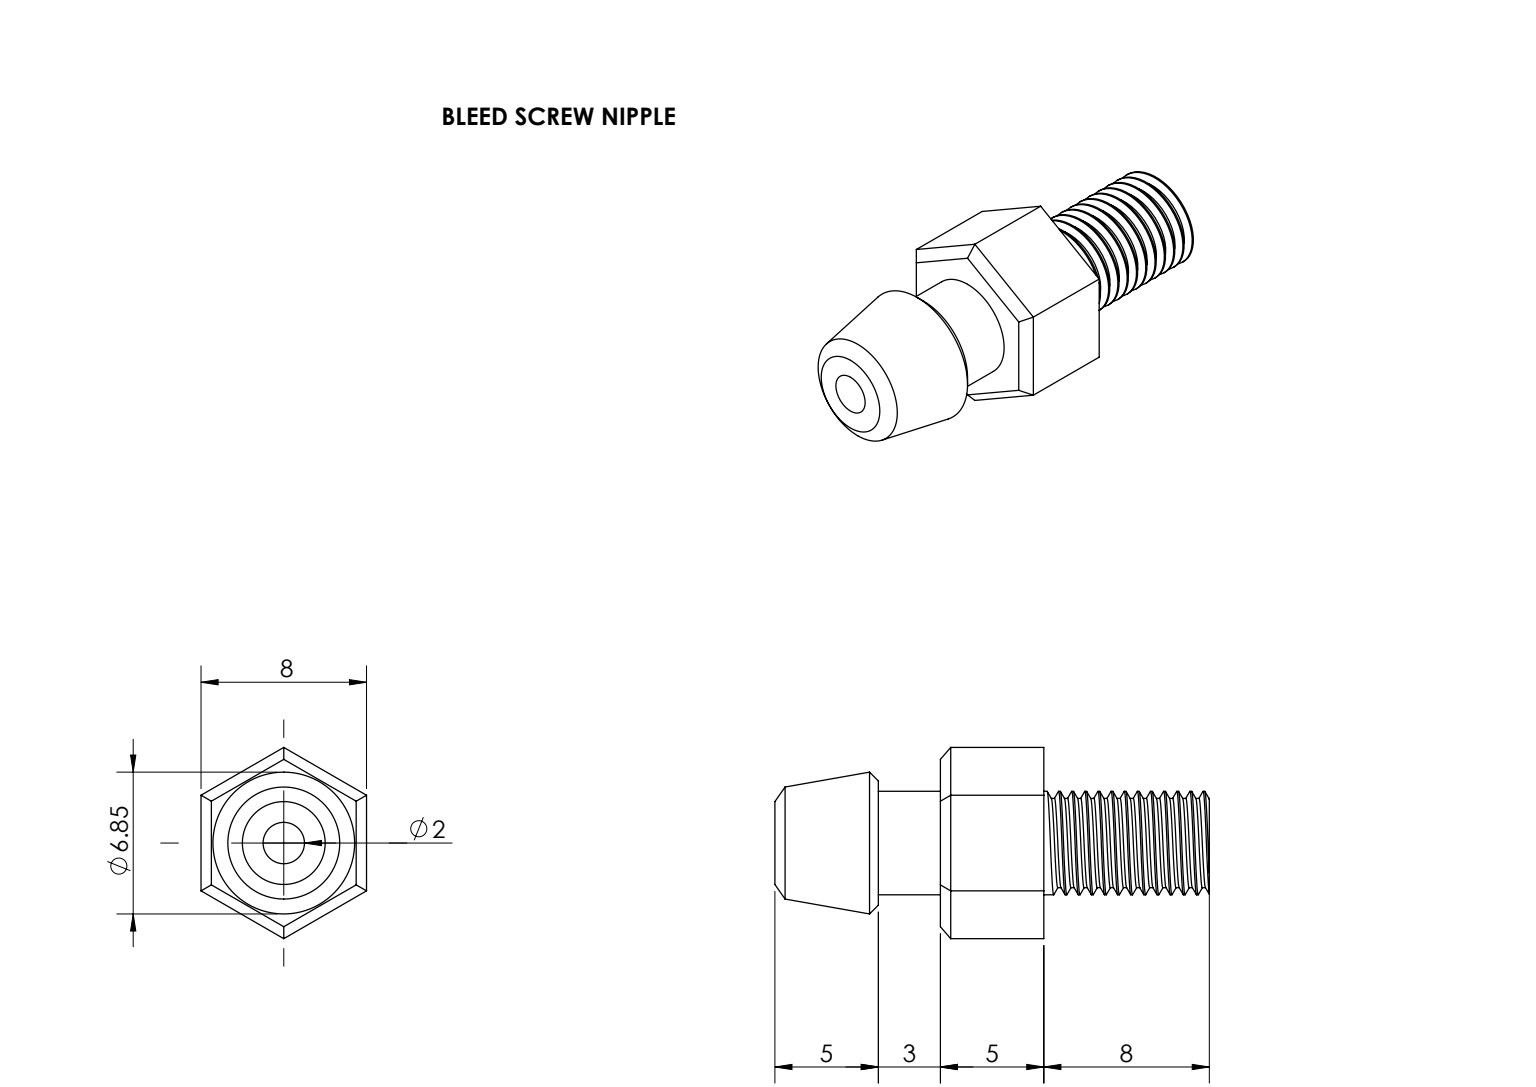
ISO-10303-21;
HEADER;
FILE_DESCRIPTION (('STEP AP214'),
    '1' );
FILE_NAME ('Bleed Screw Nipple.step',
    '2026-09-24T10:28:59',
    ( '' ),
    ( '' ),
    'SwSTEP 2.0',
    'SolidWorks 2026',
    '' );
FILE_SCHEMA (( 'AUTOMOTIVE_DESIGN' ));
ENDSEC;

DATA;
#2=CARTESIAN_POINT ( 'NONE',  ( 28.76238721243587193, -5.825490297734302381, -3.627061608673667781 ) ) ;
#3=CARTESIAN_POINT ( 'NONE',  ( 28.60033944477555323, -4.591072787911525843, -8.283357778048662468 ) ) ;
#4=FACE_OUTER_BOUND ( 'NONE', #16848, .T. ) ;
#16=CARTESIAN_POINT ( 'NONE',  ( 29.62036837594175154, -3.214238380052812261, -3.627061608673662896 ) ) ;
#18=ORIENTED_EDGE ( 'NONE', *, *, #8443, .T. ) ;
#21=CARTESIAN_POINT ( 'NONE',  ( 32.63137222500256485, -6.623491938275930302, -6.453230759126470595 ) ) ;
#34=CONICAL_SURFACE ( 'NONE', #10154, 3.500000000000004885, 0.1745329251994333364 ) ;
#35=CARTESIAN_POINT ( 'NONE',  ( 26.41562710823574278, -3.600346414165641828, -7.939653947423660263 ) ) ;
#38=ORIENTED_EDGE ( 'NONE', *, *, #3823, .T. ) ;
#44=VECTOR ( 'NONE', #8259, 1000.000000000000227 ) ;
#61=AXIS2_PLACEMENT_3D ( 'NONE', #16473, #4043, #10648 ) ;
#72=CARTESIAN_POINT ( 'NONE',  ( 25.86833963875586306, -3.039313213345869791, -4.705209693361160461 ) ) ;
#74=CARTESIAN_POINT ( 'NONE',  ( 29.12189622942009493, -1.620608325512071568, -5.783357778048658027 ) ) ;
#76=CARTESIAN_POINT ( 'NONE',  ( 31.70371634254663817, -2.036456781249897485, -4.533357778048659803 ) ) ;
#81=CARTESIAN_POINT ( 'NONE',  ( 29.62036837594175154, -3.214238380052812261, -3.627061608673662896 ) ) ;
#82=VERTEX_POINT ( 'NONE', #13166 ) ;
#84=CARTESIAN_POINT ( 'NONE',  ( 27.88665588685489993, -3.423116496867954162, -3.627061608673662008 ) ) ;
#95=CARTESIAN_POINT ( 'NONE',  ( 27.62849893492243325, -6.589071975465733644, -4.705209693361168455 ) ) ;
#97=LINE ( 'NONE', #5605, #15979 ) ;
#109=CARTESIAN_POINT ( 'NONE',  ( 26.84461768998868436, -2.294720455324902542, -5.783357778048658915 ) ) ;
#111=PLANE ( 'NONE',  #4436 ) ;
#119=ORIENTED_EDGE ( 'NONE', *, *, #5679, .T. ) ;
#123=CARTESIAN_POINT ( 'NONE',  ( 31.90644508241650357, -6.373472726347483963, -7.033357778048666908 ) ) ;
#135=ORIENTED_EDGE ( 'NONE', *, *, #7750, .F. ) ;
#150=CARTESIAN_POINT ( 'NONE',  ( 31.92138306490751987, -2.737139032229836566, -3.283357778048662023 ) ) ;
#160=CARTESIAN_POINT ( 'NONE',  ( 26.52522735095806894, -6.721994413439005278, -4.705209693361169343 ) ) ;
#161=CARTESIAN_POINT ( 'NONE',  ( 33.50243880635947846, -1.482387629897225390, -5.783357778048663356 ) ) ;
#162=CARTESIAN_POINT ( 'NONE',  ( 27.92859066579839222, -3.218191664895003967, -8.283357778048658915 ) ) ;
#166=CARTESIAN_POINT ( 'NONE',  ( 31.30154412293507349, -3.011689903141150815, -7.939653947423660263 ) ) ;
#168=CARTESIAN_POINT ( 'NONE',  ( 28.28502977505876359, -2.748149777785362957, -6.861505862736158257 ) ) ;
#179=CARTESIAN_POINT ( 'NONE',  ( 29.35841309260160159, -6.680460261459264970, -4.533357778048668685 ) ) ;
#180=CARTESIAN_POINT ( 'NONE',  ( 29.51982165028991645, -6.361204938940122844, -4.705209693361168455 ) ) ;
#191=CARTESIAN_POINT ( 'NONE',  ( 39.34669483983374505, -6.862522726337943801, -6.650911402496568314 ) ) ;
#193=CARTESIAN_POINT ( 'NONE',  ( 27.60205212784272177, -2.830435096530727446, -4.705209693361161349 ) ) ;
#195=ORIENTED_EDGE ( 'NONE', *, *, #15251, .T. ) ;
#209=CARTESIAN_POINT ( 'NONE',  ( 42.20068782821381603, -5.470578387159230616, -5.783357778048662468 ) ) ;
#212=CARTESIAN_POINT ( 'NONE',  ( 33.55383270609817714, -5.448088258586239796, -3.283357778048667797 ) ) ;
#214=CARTESIAN_POINT ( 'NONE',  ( 31.61111609099199171, -1.710254666422835745, -5.783357778048662468 ) ) ;
#220=DIRECTION ( 'NONE',  ( 0.9928203230275512992, 0.1196152422706610319, 9.614813431917826478E-17 ) ) ;
#245=ORIENTED_EDGE ( 'NONE', *, *, #2656, .T. ) ;
#247=DIRECTION ( 'NONE',  ( -0.9928203230275512992, -0.1196152422706610319, -9.614813431917826478E-17 ) ) ;
#252=CYLINDRICAL_SURFACE ( 'NONE', #8155, 1.000000000000000000 ) ;
#255=CARTESIAN_POINT ( 'NONE',  ( 31.11087420047036289, -5.742416513891037688, -3.283357778048667797 ) ) ;
#260=CARTESIAN_POINT ( 'NONE',  ( 32.77257290155422709, -2.834459985843461816, -3.627061608673662896 ) ) ;
#262=CARTESIAN_POINT ( 'NONE',  ( 25.76466184735054910, -2.811881907026620553, -6.248149982130924762 ) ) ;
#267=EDGE_LOOP ( 'NONE', ( #17915, #6076 ) ) ;
#269=DIRECTION ( 'NONE',  ( -0.1196152422706618645, 0.9928203230275510771, 0.000000000000000000 ) ) ;
#273=CARTESIAN_POINT ( 'NONE',  ( 30.04066231269008469, -3.163601260824890904, -7.939653947423660263 ) ) ;
#274=CARTESIAN_POINT ( 'NONE',  ( 29.26075783691881682, -2.330785036554694489, -4.533357778048659803 ) ) ;
#275=CARTESIAN_POINT ( 'NONE',  ( 26.01652455409633902, -4.902371455920926380, -5.783357778048663356 ) ) ;
#286=VECTOR ( 'NONE', #8460, 1000.000000000000227 ) ;
#289=CARTESIAN_POINT ( 'NONE',  ( 26.35439372113758694, -4.861664893681965083, -7.939653947423662039 ) ) ;
#296=AXIS2_PLACEMENT_3D ( 'NONE', #16194, #10362, #13007 ) ;
#305=CARTESIAN_POINT ( 'NONE',  ( 33.16732689266149237, -6.221561368663743430, -7.033357778048666908 ) ) ;
#317=VERTEX_POINT ( 'NONE', #12603 ) ;
#320=( BOUNDED_CURVE ( )  B_SPLINE_CURVE ( 2, ( #15229, #5785, #179, #16687, #11299, #4179, #6980, #13960, #12681 ),
 .UNSPECIFIED., .F., .T. ) 
 B_SPLINE_CURVE_WITH_KNOTS ( ( 3, 2, 2, 2, 3 ),
 ( 0.5192307692307692735, 0.5256410256410256610, 0.5384615384615384359, 0.5512820512820513219, 0.5576923076923077094 ),
 .UNSPECIFIED. ) 
 CURVE ( )  GEOMETRIC_REPRESENTATION_ITEM ( )  RATIONAL_B_SPLINE_CURVE ( ( 0.9330127018922192983, 0.9330127018922198534, 1.000000000000000000, 0.8660254037844387076, 1.000000000000000000, 0.8660254037844387076, 1.000000000000000000, 0.9330127018922194093, 0.9330127018922194093 ) ) 
 REPRESENTATION_ITEM ( '' )  );
#323=CARTESIAN_POINT ( 'NONE',  ( 30.17644170758179101, -4.401183590806859947, -3.283357778048664688 ) ) ;
#332=CARTESIAN_POINT ( 'NONE',  ( 32.17274868998081416, -2.279756424927169345, -4.705209693361160461 ) ) ;
#340=EDGE_CURVE ( 'NONE', #8339, #14403, #8608, .T. ) ;
#347=DIRECTION ( 'NONE',  ( 0.000000000000000000, 0.5027044994213121232, -0.8644583195629318428 ) ) ;
#348=CARTESIAN_POINT ( 'NONE',  ( 31.80137159822941939, -6.386132006154467078, -4.533357778048668685 ) ) ;
#352=CARTESIAN_POINT ( 'NONE',  ( 27.36943512155133362, -2.558652073080304845, -4.533357778048659803 ) ) ;
#356=CARTESIAN_POINT ( 'NONE',  ( 30.02326902268086428, -5.673578940050561847, -3.627061608673667781 ) ) ;
#365=ADVANCED_FACE ( 'NONE', ( #4, #13869 ), #9593, .F. ) ;
#368=DIRECTION ( 'NONE',  ( -0.1196152422706609625, 0.9928203230275510771, 0.000000000000000000 ) ) ;
#372=CARTESIAN_POINT ( 'NONE',  ( 32.91278983782564183, -5.325448745358647429, -7.939653947423664704 ) ) ;
#373=CARTESIAN_POINT ( 'NONE',  ( 30.05329989404488700, -6.934098741245490416, -5.113484796970860558 ) ) ;
#379=CARTESIAN_POINT ( 'NONE',  ( 27.82847066025702887, -2.165988739474055791, -5.783357778048658027 ) ) ;
#389=ADVANCED_FACE ( 'NONE', ( #12512 ), #15232, .T. ) ;
#397=VERTEX_POINT ( 'NONE', #1454 ) ;
#403=CARTESIAN_POINT ( 'NONE',  ( 31.59864285835955400, -2.049116061056871274, -7.033357778048658027 ) ) ;
#408=EDGE_CURVE ( 'NONE', #7873, #17484, #97, .T. ) ;
#414=ORIENTED_EDGE ( 'NONE', *, *, #10725, .T. ) ;
#416=CARTESIAN_POINT ( 'NONE',  ( 25.96530230012339757, -2.390463732198628399, -5.113484796970851676 ) ) ;
#419=EDGE_CURVE ( 'NONE', #15092, #4502, #11122, .T. ) ;
#425=CARTESIAN_POINT ( 'NONE',  ( 32.95080301609915097, -1.548848848676412260, -5.783357778048662468 ) ) ;
#430=CARTESIAN_POINT ( 'NONE',  ( 26.97161122272022382, -2.906390775372597712, -4.705209693361161349 ) ) ;
#435=CARTESIAN_POINT ( 'NONE',  ( 32.14656953781143756, -4.163822094218565972, -3.283357778048664688 ) ) ;
#444=ADVANCED_FACE ( 'NONE', ( #17342 ), #8707, .T. ) ;
#445=CARTESIAN_POINT ( 'NONE',  ( 26.20620856698912604, -7.060238655668615415, -4.533357778048668685 ) ) ;
#448=CARTESIAN_POINT ( 'NONE',  ( 32.14213199643172914, -2.910415664685331638, -3.627061608673662896 ) ) ;
#450=CARTESIAN_POINT ( 'NONE',  ( 26.16909369068367752, -6.168712907020689862, -7.925803108758818105 ) ) ;
#454=ORIENTED_EDGE ( 'NONE', *, *, #8512, .T. ) ;
#460=CARTESIAN_POINT ( 'NONE',  ( 31.43723430067123914, -2.368371383576012956, -6.861505862736158257 ) ) ;
#465=ADVANCED_FACE ( 'NONE', ( #10138 ), #11491, .T. ) ;
#472=CARTESIAN_POINT ( 'NONE',  ( 26.66961417369883591, -4.823687054261037055, -3.627061608673664672 ) ) ;
#476=CARTESIAN_POINT ( 'NONE',  ( 29.08935247050201767, -2.014077381790315702, -5.783357778048658027 ) ) ;
#478=DIRECTION ( 'NONE',  ( -0.9928203230275512992, -0.1196152422706610180, -4.006172263299093133E-17 ) ) ;
#484=CARTESIAN_POINT ( 'NONE',  ( 29.37220822929407760, -7.016156836349003001, -5.783357778048668685 ) ) ;
#486=CARTESIAN_POINT ( 'NONE',  ( 30.64556327217151122, -6.525384084031224496, -7.033357778048666908 ) ) ;
#501=EDGE_CURVE ( 'NONE', #82, #692, #8780, .T. ) ;
#503=CARTESIAN_POINT ( 'NONE',  ( 32.93470988637010066, -5.949778345213319497, -6.861505862736167138 ) ) ;
#507=( BOUNDED_CURVE ( )  B_SPLINE_CURVE ( 2, ( #5175, #2560, #10530, #5264, #17744, #16361, #6371, #3573, #10783, #16267, #2398, #10692, #11894, #3839, #3923, #14892, #17569, #16091, #9353, #8087, #9435, #1029, #2477, #3658, #6550, #13259, #14975, #2219, #753, #6472, #7999, #9265, #14724, #16177, #9179, #12067, #4913, #2307, #6279, #10440, #13356, #13535, #1109, #6634, #11800, #17378, #5089, #7825, #9096, #11986, #16000, #17474, #3740, #936, #14638, #10610, #841, #14809, #7914, #13448, #17652, #8181, #1205, #9778, #9873, #12614, #11052, #16614, #8263, #16439, #2909, #8348, #11220, #16, #4096, #9692, #16795, #1563, #2652, #4007, #4363, #12261, #6818, #9520, #5348, #15428, #3013, #11132, #15066, #12428, #10959, #5705, #13623, #13714, #12343, #1295, #2820, #6721, #17910, #6995, #17829, #5441, #5615, #15331, #2743, #10869, #13880, #16520, #9604, #15160, #193, #16701, #13795, #1376, #6901, #5529, #4275, #8441, #4190, #15240, #13977, #1467, #12523, #109, #7096, #7371, #5978, #5800, #14253, #11503, #4627, #11316, #472, #14069, #12790, #4536, #17074, #11415, #289, #15701, #16896, #10151, #5894, #7187, #15516, #4455, #10056 ),
 .UNSPECIFIED., .F., .T. ) 
 B_SPLINE_CURVE_WITH_KNOTS ( ( 3, 2, 2, 2, 2, 2, 2, 2, 2, 2, 2, 2, 2, 2, 2, 2, 2, 2, 2, 2, 2, 2, 2, 2, 2, 2, 2, 2, 2, 2, 2, 2, 2, 2, 2, 2, 2, 2, 2, 2, 2, 2, 2, 2, 2, 2, 2, 2, 2, 2, 2, 2, 2, 2, 2, 2, 2, 2, 2, 2, 2, 2, 2, 2, 2, 2, 2, 2, 2, 2, 2, 2, 2, 3 ),
 ( 0.000000000000000000, 0.01322951968774666726, 0.02645903937549333451, 0.03968855906324000177, 0.05291807875098666902, 0.06614759843873332934, 0.07937711812648000353, 0.09260663781422667773, 0.1058361575019733380, 0.1190656771897200122, 0.1322951968774666587, 0.1455247165652133190, 0.1587542362529600071, 0.1719837559407066396, 0.1852132756284533555, 0.1984427953162000158, 0.2116723150039466761, 0.2249018346916933364, 0.2381313543794400245, 0.2513608740671866570, 0.2645903937549333174, 0.2778199134426800332, 0.2910494331304266380, 0.3042789528181733538, 0.3175084725059200141, 0.3307379921936667300, 0.3439675118814132793, 0.3571970315691599951, 0.3704265512569067109, 0.3836560709446533712, 0.3968855906324000316, 0.4101151103201466364, 0.4233446300078933522, 0.4365741496956400125, 0.4498036693833866728, 0.4630331890711333331, 0.4762627087588800490, 0.4894922284466267093, 0.5027217481343733141, 0.5159512678221199744, 0.5291807875098666347, 0.5424103071976132950, 0.5556398268853600664, 0.5688693465731067267, 0.5820988662608532760, 0.5953283859485999363, 0.6085579056363467076, 0.6217874253240932569, 0.6350169450118400283, 0.6482464646995866886, 0.6614759843873334599, 0.6747055040750800092, 0.6879350237628265585, 0.7011645434505734409, 0.7143940631383199902, 0.7276235828260666505, 0.7408531025138134218, 0.7540826222015599711, 0.7673121418893067425, 0.7805416615770532918, 0.7937711812648000631, 0.8070007009525467234, 0.8202302206402932727, 0.8334597403280399330, 0.8466892600157867044, 0.8599187797035333647, 0.8731482993912800250, 0.8863778190790266853, 0.8996073387667733456, 0.9128368584545200060, 0.9260663781422666663, 0.9392958978300133266, 0.9525254175177600979, 0.9555550897579921932 ),
 .UNSPECIFIED. ) 
 CURVE ( )  GEOMETRIC_REPRESENTATION_ITEM ( )  RATIONAL_B_SPLINE_CURVE ( ( 1.000000000000000000, 0.8660254037844387076, 1.000000000000000000, 0.8660254037844387076, 1.000000000000000000, 0.8660254037844387076, 1.000000000000000000, 0.8660254037844387076, 1.000000000000000000, 0.8660254037844387076, 1.000000000000000000, 0.8660254037844387076, 1.000000000000000000, 0.8660254037844387076, 1.000000000000000000, 0.8660254037844387076, 1.000000000000000000, 0.8660254037844387076, 1.000000000000000000, 0.8660254037844387076, 1.000000000000000000, 0.8660254037844387076, 1.000000000000000000, 0.8660254037844387076, 1.000000000000000000, 0.8660254037844387076, 1.000000000000000000, 0.8660254037844387076, 1.000000000000000000, 0.8660254037844387076, 1.000000000000000000, 0.8660254037844387076, 1.000000000000000000, 0.8660254037844387076, 1.000000000000000000, 0.8660254037844387076, 1.000000000000000000, 0.8660254037844387076, 1.000000000000000000, 0.8660254037844387076, 1.000000000000000000, 0.8660254037844387076, 1.000000000000000000, 0.8660254037844387076, 1.000000000000000000, 0.8660254037844387076, 1.000000000000000000, 0.8660254037844387076, 1.000000000000000000, 0.8660254037844387076, 1.000000000000000000, 0.8660254037844387076, 1.000000000000000000, 0.8660254037844387076, 1.000000000000000000, 0.8660254037844387076, 1.000000000000000000, 0.8660254037844387076, 1.000000000000000000, 0.8660254037844387076, 1.000000000000000000, 0.8660254037844387076, 1.000000000000000000, 0.8660254037844387076, 1.000000000000000000, 0.8660254037844387076, 1.000000000000000000, 0.8660254037844387076, 1.000000000000000000, 0.8660254037844387076, 1.000000000000000000, 0.8660254037844387076, 1.000000000000000000, 0.8660254037844387076, 1.000000000000000000, 0.8660254037844387076, 1.000000000000000000, 0.8660254037844387076, 1.000000000000000000, 0.8660254037844387076, 1.000000000000000000, 0.8660254037844387076, 1.000000000000000000, 0.8660254037844387076, 1.000000000000000000, 0.8660254037844387076, 1.000000000000000000, 0.8660254037844387076, 1.000000000000000000, 0.8660254037844387076, 1.000000000000000000, 0.8660254037844387076, 1.000000000000000000, 0.8660254037844387076, 1.000000000000000000, 0.8660254037844387076, 1.000000000000000000, 0.8660254037844387076, 1.000000000000000000, 0.8660254037844387076, 1.000000000000000000, 0.8660254037844387076, 1.000000000000000000, 0.8660254037844387076, 1.000000000000000000, 0.8660254037844387076, 1.000000000000000000, 0.8660254037844387076, 1.000000000000000000, 0.8660254037844387076, 1.000000000000000000, 0.8660254037844387076, 1.000000000000000000, 0.8660254037844387076, 1.000000000000000000, 0.8660254037844387076, 1.000000000000000000, 0.8660254037844387076, 1.000000000000000000, 0.8660254037844387076, 1.000000000000000000, 0.8660254037844387076, 1.000000000000000000, 0.8660254037844387076, 1.000000000000000000, 0.8660254037844387076, 1.000000000000000000, 0.8660254037844387076, 1.000000000000000000, 0.8660254037844387076, 1.000000000000000000, 0.8660254037844387076, 1.000000000000000000, 0.8660254037844387076, 1.000000000000000000, 0.8660254037844387076, 1.000000000000000000, 0.8660254037844387076, 1.000000000000000000, 0.8660254037844387076, 1.000000000000000000, 0.8660254037844387076, 1.000000000000000000, 0.8660254037844387076, 1.000000000000000000, 0.9693186809021840933, 0.9526899265169710418 ) ) 
 REPRESENTATION_ITEM ( '' )  );
#511=CARTESIAN_POINT ( 'NONE',  ( 26.49461065740898036, -7.352653653197164019, -5.783357778048668685 ) ) ;
#519=ORIENTED_EDGE ( 'NONE', *, *, #4015, .F. ) ;
#520=CARTESIAN_POINT ( 'NONE',  ( 26.31065902414478686, -7.328232685206446106, -6.312034385895062272 ) ) ;
#522=CARTESIAN_POINT ( 'NONE',  ( 26.69778786461289855, -6.274106265784127778, -3.283357778048667797 ) ) ;
#527=CARTESIAN_POINT ( 'NONE',  ( 27.73357241910951743, -6.576412695658750529, -6.861505862736166250 ) ) ;
#529=CARTESIAN_POINT ( 'NONE',  ( 25.99533317148741318, -3.650983533393564517, -3.627061608673662008 ) ) ;
#541=CARTESIAN_POINT ( 'NONE',  ( 33.13163345120441505, -4.045141346131868154, -3.627061608673664672 ) ) ;
#542=DIRECTION ( 'NONE',  ( -0.1196152422706610735, 0.9928203230275511881, 0.000000000000000000 ) ) ;
#551=CARTESIAN_POINT ( 'NONE',  ( 30.88568772756644520, -4.315733451902305617, -3.283357778048664688 ) ) ;
#554=ORIENTED_EDGE ( 'NONE', *, *, #8603, .F. ) ;
#555=CYLINDRICAL_SURFACE ( 'NONE', #10636, 2.500000000000001776 ) ;
#564=ORIENTED_EDGE ( 'NONE', *, *, #6190, .F. ) ;
#567=VECTOR ( 'NONE', #13806, 1000.000000000000227 ) ;
#574=CARTESIAN_POINT ( 'NONE',  ( 27.65467808709180630, -4.705006306174339237, -3.283357778048664688 ) ) ;
#576=DIRECTION ( 'NONE',  ( -0.9928203230275510771, -0.1196152422706614760, -0.000000000000000000 ) ) ;
#580=CARTESIAN_POINT ( 'NONE',  ( 26.31065902414478330, -7.328232685206446106, -6.312034385895062272 ) ) ;
#583=DIRECTION ( 'NONE',  ( 0.9928203230275510771, 0.1196152422706610596, 9.614813431917826478E-17 ) ) ;
#586=PLANE ( 'NONE',  #16874 ) ;
#588=CARTESIAN_POINT ( 'NONE',  ( 29.81239362717914787, -2.264323817775507397, -4.533357778048659803 ) ) ;
#590=LINE ( 'NONE', #17666, #6969 ) ;
#595=CARTESIAN_POINT ( 'NONE',  ( 33.24613200752366282, -6.212066908601060256, -7.033357778048666908 ) ) ;
#609=ORIENTED_EDGE ( 'NONE', *, *, #13028, .F. ) ;
#612=FACE_OUTER_BOUND ( 'NONE', #16099, .T. ) ;
#616=CARTESIAN_POINT ( 'NONE',  ( 33.17094678975809074, -2.159493266760871499, -6.861505862736159145 ) ) ;
#620=CARTESIAN_POINT ( 'NONE',  ( 28.98992747081925359, -3.290194058894681639, -3.627061608673662896 ) ) ;
#627=VERTEX_POINT ( 'NONE', #4279 ) ;
#632=CARTESIAN_POINT ( 'NONE',  ( 33.43363050022580296, -2.127845067243429256, -4.705209693361160461 ) ) ;
#641=ORIENTED_EDGE ( 'NONE', *, *, #16806, .F. ) ;
#645=CARTESIAN_POINT ( 'NONE',  ( 31.34233605952372415, -6.778795339760710803, -5.783357778048663356 ) ) ;
#652=ORIENTED_EDGE ( 'NONE', *, *, #11187, .T. ) ;
#655=CARTESIAN_POINT ( 'NONE',  ( 29.97449477918272009, -6.943593201308171814, -5.113484796970856117 ) ) ;
#663=CARTESIAN_POINT ( 'NONE',  ( 26.31556265977298992, -7.384422263489805793, -5.783357778048663356 ) ) ;
#664=CARTESIAN_POINT ( 'NONE',  ( 27.15176839919044482, -1.857969822100365098, -5.783357778048658027 ) ) ;
#670=CARTESIAN_POINT ( 'NONE',  ( 30.45035428628836627, -2.914368949527523789, -8.283357778048660691 ) ) ;
#685=CARTESIAN_POINT ( 'NONE',  ( 30.60986983071443390, -4.348964061499348333, -3.627061608673664672 ) ) ;
#692=VERTEX_POINT ( 'NONE', #9969 ) ;
#693=CARTESIAN_POINT ( 'NONE',  ( 27.50150540219088313, -5.977401655418042914, -3.627061608673667781 ) ) ;
#699=ORIENTED_EDGE ( 'NONE', *, *, #2456, .F. ) ;
#704=CARTESIAN_POINT ( 'NONE',  ( 33.38562051666750818, -5.268481986227246061, -7.939653947423664704 ) ) ;
#707=CARTESIAN_POINT ( 'NONE',  ( 27.93049598394382116, -4.671775696577297410, -3.627061608673664672 ) ) ;
#711=CARTESIAN_POINT ( 'NONE',  ( 32.69820532807177216, -4.097360875439379768, -3.283357778048664688 ) ) ;
#721=CARTESIAN_POINT ( 'NONE',  ( 32.06767520579373354, -2.292415704734142690, -6.861505862736158257 ) ) ;
#726=CARTESIAN_POINT ( 'NONE',  ( 31.32102116884452414, -5.717097954277069682, -8.283357778048664244 ) ) ;
#731=CARTESIAN_POINT ( 'NONE',  ( 33.76207435632690590, -3.969185667289998332, -3.627061608673664672 ) ) ;
#751=CARTESIAN_POINT ( 'NONE',  ( 26.52132749406794687, -1.933925500942234921, -5.783357778048658027 ) ) ;
#753=CARTESIAN_POINT ( 'NONE',  ( 31.91006497951310550, -2.311404624444611589, -6.861505862736159145 ) ) ;
#757=VERTEX_POINT ( 'NONE', #7191 ) ;
#771=CARTESIAN_POINT ( 'NONE',  ( 31.65190802758064592, -5.477360103042387074, -7.939653947423664704 ) ) ;
#778=EDGE_LOOP ( 'NONE', ( #8349, #2601, #9455, #8775 ) ) ;
#781=CARTESIAN_POINT ( 'NONE',  ( 31.26353094466156080, -6.788289799823394866, -5.783357778048663356 ) ) ;
#785=EDGE_CURVE ( 'NONE', #4502, #14075, #17606, .T. ) ;
#789=CARTESIAN_POINT ( 'NONE',  ( 31.91459173804834748, -5.445711903524953712, -3.627061608673667781 ) ) ;
#793=CARTESIAN_POINT ( 'NONE',  ( 28.23249303296521617, -2.754479417688857179, -4.705209693361161349 ) ) ;
#806=CARTESIAN_POINT ( 'NONE',  ( 29.55043834383899437, -5.730545699181964991, -3.627061608673668225 ) ) ;
#808=CARTESIAN_POINT ( 'NONE',  ( 32.61569110240115776, -6.288022587442930522, -7.033357778048666908 ) ) ;
#809=CARTESIAN_POINT ( 'NONE',  ( 31.34233605952372415, -6.778795339760710803, -5.783357778048663356 ) ) ;
#814=CARTESIAN_POINT ( 'NONE',  ( 33.33308377457396432, -5.274811626130743392, -3.627061608673668225 ) ) ;
#823=AXIS2_PLACEMENT_3D ( 'NONE', #191, #1650, #1838 ) ;
#829=EDGE_CURVE ( 'NONE', #397, #17258, #16253, .T. ) ;
#840=CARTESIAN_POINT ( 'NONE',  ( 28.64916707261694384, -6.765910400363817523, -4.533357778048668685 ) ) ;
#841=CARTESIAN_POINT ( 'NONE',  ( 30.88577694472199298, -6.196634301449400084, -6.861505862736166250 ) ) ;
#844=CARTESIAN_POINT ( 'NONE',  ( 26.66770885555339987, -3.370103022578743612, -8.283357778048660691 ) ) ;
#852=CARTESIAN_POINT ( 'NONE',  ( 29.79859849048667897, -1.928627242885762705, -5.783357778048664244 ) ) ;
#855=CYLINDRICAL_SURFACE ( 'NONE', #296, 2.500000000000001776 ) ;
#860=CARTESIAN_POINT ( 'NONE',  ( 30.40841950734487753, -3.119293781500474427, -3.627061608673662008 ) ) ;
#862=CARTESIAN_POINT ( 'NONE',  ( 26.18940075748478691, -6.337263906362392341, -7.823530922983556124 ) ) ;
#873=CARTESIAN_POINT ( 'NONE',  ( 32.89331279191618762, -2.620040694222726785, -8.283357778048660691 ) ) ;
#874=FACE_OUTER_BOUND ( 'NONE', #5971, .T. ) ;
#875=EDGE_CURVE ( 'NONE', #17192, #6885, #1465, .T. ) ;
#876=CARTESIAN_POINT ( 'NONE',  ( 28.20260476654369697, -6.819712339336020612, -7.033357778048666908 ) ) ;
#880=CARTESIAN_POINT ( 'NONE',  ( 32.67202617590239555, -5.981426544730773287, -4.705209693361168455 ) ) ;
#882=CARTESIAN_POINT ( 'NONE',  ( 31.98525019727866692, -6.363978266284800789, -7.033357778048666908 ) ) ;
#884=CARTESIAN_POINT ( 'NONE',  ( 26.97161122272022382, -2.906390775372597712, -4.705209693361161349 ) ) ;
#887=CARTESIAN_POINT ( 'NONE',  ( 33.15485366002904755, -6.560422763297783177, -5.783357778048663356 ) ) ;
#890=ORIENTED_EDGE ( 'NONE', *, *, #2202, .F. ) ;
#899=DIRECTION ( 'NONE',  ( 0.9928203230275510771, 0.1196152422706610596, 9.614813431917826478E-17 ) ) ;
#901=CARTESIAN_POINT ( 'NONE',  ( 30.39102621733566423, -5.629271460726126719, -7.939653947423664704 ) ) ;
#902=CARTESIAN_POINT ( 'NONE',  ( 30.32207992551315812, -1.865558067907615802, -6.453230759126468818 ) ) ;
#911=CARTESIAN_POINT ( 'NONE',  ( 32.19919549706052209, -6.038393303862174655, -4.705209693361169343 ) ) ;
#918=CARTESIAN_POINT ( 'NONE',  ( 32.77701044293393551, -4.087866415376695706, -3.283357778048664688 ) ) ;
#921=EDGE_LOOP ( 'NONE', ( #12504, #6661, #5208, #15907 ) ) ;
#930=VECTOR ( 'NONE', #8401, 1000.000000000000227 ) ;
#934=CARTESIAN_POINT ( 'NONE',  ( 28.15758777499317489, -7.552042790248305160, -5.783357778048669573 ) ) ;
#936=CARTESIAN_POINT ( 'NONE',  ( 30.67110321781257909, -3.087645581983020637, -7.939653947423660263 ) ) ;
#949=DIRECTION ( 'NONE',  ( -0.9928203230275512992, -0.1196152422706610180, -4.006172263299093133E-17 ) ) ;
#956=CARTESIAN_POINT ( 'NONE',  ( 28.71854711534694715, -4.576831098024959132, -3.627061608673664672 ) ) ;
#957=CARTESIAN_POINT ( 'NONE',  ( 33.19286683830256379, -2.783822866615540903, -7.939653947423660263 ) ) ;
#967=LINE ( 'NONE', #8942, #11342 ) ;
#972=CARTESIAN_POINT ( 'NONE',  ( 39.14763340350798160, -5.210289818862206879, -9.533357778048658915 ) ) ;
#976=CARTESIAN_POINT ( 'NONE',  ( 32.01513846370018967, -2.298745344637636912, -4.705209693361161349 ) ) ;
#983=CARTESIAN_POINT ( 'NONE',  ( 29.08935247050201767, -2.014077381790315702, -5.783357778048658027 ) ) ;
#988=VECTOR ( 'NONE', #8852, 1000.000000000000227 ) ;
#989=ORIENTED_EDGE ( 'NONE', *, *, #10188, .F. ) ;
#998=CARTESIAN_POINT ( 'NONE',  ( 30.92509028327567933, -4.310986222078405206, -7.939653947423662039 ) ) ;
#1000=CARTESIAN_POINT ( 'NONE',  ( 31.15208055228630357, -2.102918000029084578, -4.533357778048659803 ) ) ;
#1006=CARTESIAN_POINT ( 'NONE',  ( 33.44685390376565692, -4.007163506710925027, -7.939653947423662039 ) ) ;
#1027=( BOUNDED_CURVE ( )  B_SPLINE_CURVE ( 2, ( #17419, #3613, #12020, #14762, #14674, #2255, #882, #9215, #13397 ),
 .UNSPECIFIED., .F., .T. ) 
 B_SPLINE_CURVE_WITH_KNOTS ( ( 3, 2, 2, 2, 3 ),
 ( 0.1730769230769231004, 0.1794871794871794879, 0.1923076923076923184, 0.2051282051282051211, 0.2115384615384615641 ),
 .UNSPECIFIED. ) 
 CURVE ( )  GEOMETRIC_REPRESENTATION_ITEM ( )  RATIONAL_B_SPLINE_CURVE ( ( 0.9330127018922194093, 0.9330127018922196314, 1.000000000000000000, 0.8660254037844387076, 1.000000000000000000, 0.8660254037844387076, 1.000000000000000000, 0.9330127018922190762, 0.9330127018922194093 ) ) 
 REPRESENTATION_ITEM ( '' )  );
#1028=DIRECTION ( 'NONE',  ( 1.000000000000000000, 0.000000000000000000, -0.000000000000000000 ) ) ;
#1029=CARTESIAN_POINT ( 'NONE',  ( 32.79901970863393501, -6.593096864778464017, -5.783357778048668685 ) ) ;
#1038=EDGE_CURVE ( 'NONE', #4277, #15625, #10962, .T. ) ;
#1039=CARTESIAN_POINT ( 'NONE',  ( 32.32036211097666012, -1.624804527518282748, -5.783357778048663356 ) ) ;
#1044=CARTESIAN_POINT ( 'NONE',  ( 29.14753769709988518, -3.271205139184214516, -3.627061608673662008 ) ) ;
#1057=CARTESIAN_POINT ( 'NONE',  ( 28.04870365451522218, -4.657534006690712935, -8.283357778048662468 ) ) ;
#1067=ORIENTED_EDGE ( 'NONE', *, *, #5837, .F. ) ;
#1068=ORIENTED_EDGE ( 'NONE', *, *, #3042, .T. ) ;
#1071=DIRECTION ( 'NONE',  ( 0.9928203230275512992, 0.1196152422706610041, 9.614813431917824012E-17 ) ) ;
#1076=CARTESIAN_POINT ( 'NONE',  ( 31.04338717100262102, -6.177645381738930297, -6.861505862736167138 ) ) ;
#1078=CARTESIAN_POINT ( 'NONE',  ( 31.83134908525019213, -4.201799933639492224, -8.283357778048662468 ) ) ;
#1085=CARTESIAN_POINT ( 'NONE',  ( 32.93018312783485868, -2.815471066132993805, -3.627061608673662008 ) ) ;
#1087=EDGE_CURVE ( 'NONE', #17201, #15670, #17322, .T. ) ;
#1088=CARTESIAN_POINT ( 'NONE',  ( 30.42903939560917337, -1.852671564043892660, -5.783357778048658027 ) ) ;
#1090=( BOUNDED_CURVE ( )  B_SPLINE_CURVE ( 2, ( #14792, #14707, #2289, #10422, #918, #9082, #10592, #14623, #11605 ),
 .UNSPECIFIED., .F., .T. ) 
 B_SPLINE_CURVE_WITH_KNOTS ( ( 3, 2, 2, 2, 3 ),
 ( 0.05769230769230770939, 0.06410256410256409687, 0.07692307692307692735, 0.08974358974358974395, 0.09615384615384617306 ),
 .UNSPECIFIED. ) 
 CURVE ( )  GEOMETRIC_REPRESENTATION_ITEM ( )  RATIONAL_B_SPLINE_CURVE ( ( 0.9330127018922194093, 0.9330127018922196314, 1.000000000000000000, 0.8660254037844387076, 1.000000000000000000, 0.8660254037844387076, 1.000000000000000000, 0.9330127018922191873, 0.9330127018922194093 ) ) 
 REPRESENTATION_ITEM ( '' )  );
#1105=DIRECTION ( 'NONE',  ( 0.9928203230275510771, 0.1196152422706609902, 4.006172263299092517E-17 ) ) ;
#1109=CARTESIAN_POINT ( 'NONE',  ( 31.39792096211754924, -4.254019462947003838, -7.939653947423662039 ) ) ;
#1110=( BOUNDED_CURVE ( )  B_SPLINE_CURVE ( 2, ( #15566, #14564, #348, #6199, #6287, #14645, #7660, #11809, #13269 ),
 .UNSPECIFIED., .F., .T. ) 
 B_SPLINE_CURVE_WITH_KNOTS ( ( 3, 2, 2, 2, 3 ),
 ( 0.2884615384615384914, 0.2948717948717948789, 0.3076923076923077094, 0.3205128205128205399, 0.3269230769230769273 ),
 .UNSPECIFIED. ) 
 CURVE ( )  GEOMETRIC_REPRESENTATION_ITEM ( )  RATIONAL_B_SPLINE_CURVE ( ( 0.9330127018922194093, 0.9330127018922196314, 1.000000000000000000, 0.8660254037844387076, 1.000000000000000000, 0.8660254037844387076, 1.000000000000000000, 0.9330127018922194093, 0.9330127018922194093 ) ) 
 REPRESENTATION_ITEM ( '' )  );
#1125=CARTESIAN_POINT ( 'NONE',  ( 27.78610916120306129, -6.570083055755264745, -4.705209693361169343 ) ) ;
#1129=EDGE_CURVE ( 'NONE', #4586, #7873, #17252, .T. ) ;
#1163=CARTESIAN_POINT ( 'NONE',  ( 28.83304567166618781, -6.743756660494150346, -7.033357778048666908 ) ) ;
#1167=DIRECTION ( 'NONE',  ( 0.9928203230275510771, 0.1196152422706609902, 4.006172263299092517E-17 ) ) ;
#1170=CARTESIAN_POINT ( 'NONE',  ( 26.20438954464326287, -6.461672570559207074, -7.734911333299593572 ) ) ;
#1173=CARTESIAN_POINT ( 'NONE',  ( 31.95146207396702565, -5.641142275435198528, -8.283357778048662468 ) ) ;
#1174=CYLINDRICAL_SURFACE ( 'NONE', #14258, 2.500000000000001776 ) ;
#1177=SURFACE_SIDE_STYLE ('',( #3895 ) ) ;
#1179=VECTOR ( 'NONE', #10787, 1000.000000000000114 ) ;
#1180=CARTESIAN_POINT ( 'NONE',  ( 30.18087924896149588, -5.654590020340094725, -3.627061608673668225 ) ) ;
#1205=CARTESIAN_POINT ( 'NONE',  ( 30.12381574833269937, -2.526612381163247267, -4.705209693361161349 ) ) ;
#1206=VECTOR ( 'NONE', #4523, 1000.000000000000227 ) ;
#1226=CARTESIAN_POINT ( 'NONE',  ( 25.88156304229571703, -4.918631652813365562, -7.939653947423662039 ) ) ;
#1227=AXIS2_PLACEMENT_3D ( 'NONE', #5967, #9955, #14335 ) ;
#1234=CARTESIAN_POINT ( 'NONE',  ( 31.61111609099199171, -1.710254666422835745, -5.783357778048661579 ) ) ;
#1266=CARTESIAN_POINT ( 'NONE',  ( 28.04870365451522218, -4.657534006690712935, -8.283357778048662468 ) ) ;
#1273=CARTESIAN_POINT ( 'NONE',  ( 27.65911562847151117, -5.958412735707574015, -3.627061608673668225 ) ) ;
#1276=CARTESIAN_POINT ( 'NONE',  ( 33.60446413004628141, -3.988174587000466342, -3.627061608673664672 ) ) ;
#1282=CARTESIAN_POINT ( 'NONE',  ( 28.87615734162756453, -4.557842178314484016, -7.939653947423662039 ) ) ;
#1294=CARTESIAN_POINT ( 'NONE',  ( 25.89088658894545603, -2.009881179784104965, -5.783357778048658027 ) ) ;
#1295=CARTESIAN_POINT ( 'NONE',  ( 28.76238721243587548, -5.825490297734302381, -3.627061608673667781 ) ) ;
#1296=EDGE_CURVE ( 'NONE', #16733, #3360, #5319, .T. ) ;
#1300=ORIENTED_EDGE ( 'NONE', *, *, #4267, .T. ) ;
#1305=EDGE_CURVE ( 'NONE', #3946, #4809, #15975, .T. ) ;
#1309=CARTESIAN_POINT ( 'NONE',  ( 26.39823381822651882, -6.110324093391315436, -3.627061608673668225 ) ) ;
#1310=DIRECTION ( 'NONE',  ( -0.1196152422706598106, 0.9928203230275514102, 0.000000000000000000 ) ) ;
#1341=CARTESIAN_POINT ( 'NONE',  ( 25.96861057204955259, -6.167300557297518360, -7.540293452860097112 ) ) ;
#1343=CARTESIAN_POINT ( 'NONE',  ( 29.94002636988270538, -4.429666970165102136, -8.283357778048662468 ) ) ;
#1345=EDGE_CURVE ( 'NONE', #15092, #16712, #4429, .T. ) ;
#1349=CARTESIAN_POINT ( 'NONE',  ( 29.15206445563513071, -6.405512418264540209, -6.861505862736167138 ) ) ;
#1361=CARTESIAN_POINT ( 'NONE',  ( 42.26049544934917179, -5.966988548673008097, -5.783357778048662468 ) ) ;
#1362=CARTESIAN_POINT ( 'NONE',  ( 30.13703915187255689, -4.405930820630744371, -7.939653947423662039 ) ) ;
#1363=CARTESIAN_POINT ( 'NONE',  ( 26.10855331130634127, -2.710563430764044490, -4.533357778048659803 ) ) ;
#1376=CARTESIAN_POINT ( 'NONE',  ( 27.51889869220010354, -3.467423976192371526, -7.939653947423660263 ) ) ;
#1394=CARTESIAN_POINT ( 'NONE',  ( 27.12922144900085186, -2.887401855662130146, -4.705209693361160461 ) ) ;
#1404=CARTESIAN_POINT ( 'NONE',  ( 27.65467808709180630, -4.705006306174339237, -3.283357778048664688 ) ) ;
#1432=AXIS2_PLACEMENT_3D ( 'NONE', #7668, #3492, #9023 ) ;
#1434=CARTESIAN_POINT ( 'NONE',  ( 29.49727470010032704, -7.390636972501882340, -5.783357778048669573 ) ) ;
#1440=CARTESIAN_POINT ( 'NONE',  ( 28.52162355051263987, -6.481468097106410475, -6.861505862736167138 ) ) ;
#1450=VECTOR ( 'NONE', #4216, 1000.000000000000000 ) ;
#1452=CARTESIAN_POINT ( 'NONE',  ( 27.71165237056504438, -5.952083095804076684, -7.939653947423664704 ) ) ;
#1454=CARTESIAN_POINT ( 'NONE',  ( 31.89397184978405519, -6.712334120981523711, -5.783357778048663356 ) ) ;
#1457=( BOUNDED_CURVE ( )  B_SPLINE_CURVE ( 2, ( #731, #9330, #13429, #17547, #7893, #9075, #1006, #2458, #11869, #7978, #13514, #814, #17719, #1085, #10509, #14524, #14618, #11777, #7631, #6609, #5240, #15876, #3639, #12139, #7801, #3451, #5067, #7711, #16154, #2107, #6346, #8980, #13152, #16070, #911, #17350, #4887, #10587, #6258, #10417, #3717, #9241, #14787, #2376, #15976, #3544, #17448, #2198, #6531, #11964, #14700, #4982, #13237, #9161, #2282, #12045, #13331, #6445, #17632, #5150, #10669, #16244, #16587, #16338, #12498, #2719, #8240, #13597, #17887, #12589, #3897, #1180, #17807, #5325, #9752, #12235, #10761, #16496, #2885, #13773, #9414, #15039, #9498, #6698, #11481, #13945, #10849, #4169, #7072, #8154, #6968, #16417, #1349, #8412, #13851, #9668, #15216, #5503, #2796, #2533, #168, #11025, #8321, #15305, #1440, #5415, #11108, #13687, #12321, #84, #3982, #2628, #4070, #5591, #16678, #4251, #1539, #14953, #8061, #1273, #6872, #6793, #10930, #9578, #15133, #12403, #14043, #3340, #7160, #12670, #6044, #15576, #15400, #9940, #11287, #1814, #8871, #8591, #16956, #10217, #3073, #1717, #8694, #3155, #4599, #529, #1629, #14222, #262 ),
 .UNSPECIFIED., .F., .T. ) 
 B_SPLINE_CURVE_WITH_KNOTS ( ( 3, 2, 2, 2, 2, 2, 2, 2, 2, 2, 2, 2, 2, 2, 2, 2, 2, 2, 2, 2, 2, 2, 2, 2, 2, 2, 2, 2, 2, 2, 2, 2, 2, 2, 2, 2, 2, 2, 2, 2, 2, 2, 2, 2, 2, 2, 2, 2, 2, 2, 2, 2, 2, 2, 2, 2, 2, 2, 2, 2, 2, 2, 2, 2, 2, 2, 2, 2, 2, 2, 2, 2, 2, 2, 3 ),
 ( 0.000000000000000000, 0.01322951878407230102, 0.02645903756814460203, 0.03968855635221691519, 0.05291807513628920406, 0.06614759392036151375, 0.07937711270443383038, 0.09260663148850611925, 0.1058361502725784081, 0.1190656690566507248, 0.1322951878407230275, 0.1455247066247953303, 0.1587542254088676608, 0.1719837441929399358, 0.1852132629770122385, 0.1984427817610845690, 0.2116723005451568163, 0.2249018193292291468, 0.2381313381133014495, 0.2513608568973737523, 0.2645903756814460550, 0.2778198944655183578, 0.2910494132495906605, 0.3042789320336629633, 0.3175084508177353215, 0.3307379696018076243, 0.3439674883858798715, 0.3571970071699521743, 0.3704265259540244770, 0.3836560447380968353, 0.3968855635221691380, 0.4101150823062413853, 0.4233446010903136325, 0.4365741198743859908, 0.4498036386584582935, 0.4630331574425305963, 0.4762626762266028990, 0.4894921950106752018, 0.5027217137947475045, 0.5159512325788198073, 0.5291807513628921100, 0.5424102701469644128, 0.5556397889310367155, 0.5688693077151090183, 0.5820988264991813210, 0.5953283452832536238, 0.6085578640673259265, 0.6217873828513982293, 0.6350169016354706431, 0.6482464204195428348, 0.6614759392036152486, 0.6747054579876874403, 0.6879349767717597430, 0.7011644955558321568, 0.7143940143399043485, 0.7276235331239767623, 0.7408530519080489540, 0.7540825706921212568, 0.7673120894761936706, 0.7805416082602658623, 0.7937711270443382761, 0.8070006458284105788, 0.8202301646124827705, 0.8334596833965551843, 0.8466892021806272650, 0.8599187209646996788, 0.8731482397487719815, 0.8863777585328441733, 0.8996072773169165870, 0.9128367961009887788, 0.9260663148850611925, 0.9392958336691334953, 0.9525253524532057980, 0.9657548712372781008, 0.9750618896629086318 ),
 .UNSPECIFIED. ) 
 CURVE ( )  GEOMETRIC_REPRESENTATION_ITEM ( )  RATIONAL_B_SPLINE_CURVE ( ( 1.000000000000000000, 0.8660254037844387076, 1.000000000000000000, 0.8660254037844387076, 1.000000000000000000, 0.8660254037844387076, 1.000000000000000000, 0.8660254037844387076, 1.000000000000000000, 0.8660254037844387076, 1.000000000000000000, 0.8660254037844387076, 1.000000000000000000, 0.8660254037844387076, 1.000000000000000000, 0.8660254037844387076, 1.000000000000000000, 0.8660254037844387076, 1.000000000000000000, 0.8660254037844387076, 1.000000000000000000, 0.8660254037844387076, 1.000000000000000000, 0.8660254037844387076, 1.000000000000000000, 0.8660254037844387076, 1.000000000000000000, 0.8660254037844387076, 1.000000000000000000, 0.8660254037844387076, 1.000000000000000000, 0.8660254037844387076, 1.000000000000000000, 0.8660254037844387076, 1.000000000000000000, 0.8660254037844387076, 1.000000000000000000, 0.8660254037844387076, 1.000000000000000000, 0.8660254037844387076, 1.000000000000000000, 0.8660254037844387076, 1.000000000000000000, 0.8660254037844387076, 1.000000000000000000, 0.8660254037844387076, 1.000000000000000000, 0.8660254037844387076, 1.000000000000000000, 0.8660254037844387076, 1.000000000000000000, 0.8660254037844387076, 1.000000000000000000, 0.8660254037844387076, 1.000000000000000000, 0.8660254037844387076, 1.000000000000000000, 0.8660254037844387076, 1.000000000000000000, 0.8660254037844387076, 1.000000000000000000, 0.8660254037844387076, 1.000000000000000000, 0.8660254037844387076, 1.000000000000000000, 0.8660254037844387076, 1.000000000000000000, 0.8660254037844387076, 1.000000000000000000, 0.8660254037844387076, 1.000000000000000000, 0.8660254037844387076, 1.000000000000000000, 0.8660254037844387076, 1.000000000000000000, 0.8660254037844387076, 1.000000000000000000, 0.8660254037844387076, 1.000000000000000000, 0.8660254037844387076, 1.000000000000000000, 0.8660254037844387076, 1.000000000000000000, 0.8660254037844387076, 1.000000000000000000, 0.8660254037844387076, 1.000000000000000000, 0.8660254037844387076, 1.000000000000000000, 0.8660254037844387076, 1.000000000000000000, 0.8660254037844387076, 1.000000000000000000, 0.8660254037844387076, 1.000000000000000000, 0.8660254037844387076, 1.000000000000000000, 0.8660254037844387076, 1.000000000000000000, 0.8660254037844387076, 1.000000000000000000, 0.8660254037844387076, 1.000000000000000000, 0.8660254037844387076, 1.000000000000000000, 0.8660254037844387076, 1.000000000000000000, 0.8660254037844387076, 1.000000000000000000, 0.8660254037844387076, 1.000000000000000000, 0.8660254037844387076, 1.000000000000000000, 0.8660254037844387076, 1.000000000000000000, 0.8660254037844387076, 1.000000000000000000, 0.8660254037844387076, 1.000000000000000000, 0.8660254037844387076, 1.000000000000000000, 0.8660254037844387076, 1.000000000000000000, 0.8660254037844387076, 1.000000000000000000, 0.8660254037844387076, 1.000000000000000000, 0.8660254037844387076, 1.000000000000000000, 0.8660254037844387076, 1.000000000000000000, 0.8660254037844387076, 1.000000000000000000, 0.8660254037844387076, 1.000000000000000000, 0.8660254037844387076, 1.000000000000000000, 0.8660254037844387076, 1.000000000000000000, 0.8660254037844387076, 1.000000000000000000, 0.8660254037844387076, 1.000000000000000000, 0.8660254037844387076, 1.000000000000000000, 0.8660254037844387076, 1.000000000000000000, 0.9057483453558528019, 0.9441095091726994237 ) ) 
 REPRESENTATION_ITEM ( '' )  );
#1458=ORIENTED_EDGE ( 'NONE', *, *, #501, .T. ) ;
#1465=( BOUNDED_CURVE ( )  B_SPLINE_CURVE ( 2, ( #17730, #2809, #16350, #3912, #3, #3993, #3826, #14962, #8072 ),
 .UNSPECIFIED., .F., .T. ) 
 B_SPLINE_CURVE_WITH_KNOTS ( ( 3, 2, 2, 2, 3 ),
 ( 0.6346153846153846922, 0.6410256410256410797, 0.6538461538461538547, 0.6666666666666666297, 0.6730769230769231282 ),
 .UNSPECIFIED. ) 
 CURVE ( )  GEOMETRIC_REPRESENTATION_ITEM ( )  RATIONAL_B_SPLINE_CURVE ( ( 0.9330127018922192983, 0.9330127018922198534, 1.000000000000000000, 0.8660254037844387076, 1.000000000000000000, 0.8660254037844387076, 1.000000000000000000, 0.9330127018922187432, 0.9330127018922192983 ) ) 
 REPRESENTATION_ITEM ( '' )  );
#1467=CARTESIAN_POINT ( 'NONE',  ( 27.09860475545177039, -3.518061095420291995, -3.627061608673662896 ) ) ;
#1476=AXIS2_PLACEMENT_3D ( 'NONE', #275, #4265, #2811 ) ;
#1483=AXIS2_PLACEMENT_3D ( 'NONE', #10857, #17729, #3824 ) ;
#1488=CARTESIAN_POINT ( 'NONE',  ( 27.15566825608056689, -6.646038734597135011, -4.705209693361169343 ) ) ;
#1490=ORIENTED_EDGE ( 'NONE', *, *, #4667, .T. ) ;
#1500=ORIENTED_EDGE ( 'NONE', *, *, #875, .F. ) ;
#1501=CARTESIAN_POINT ( 'NONE',  ( 27.19802975513453092, -2.241944418315925613, -5.783357778048658027 ) ) ;
#1521=EDGE_LOOP ( 'NONE', ( #1490, #9810 ) ) ;
#1524=ORIENTED_EDGE ( 'NONE', *, *, #10273, .T. ) ;
#1529=LINE ( 'NONE', #13842, #930 ) ;
#1530=CARTESIAN_POINT ( 'NONE',  ( 26.65222088368961195, -7.333664733486695120, -5.783357778048669573 ) ) ;
#1532=CARTESIAN_POINT ( 'NONE',  ( 28.58911057998038530, -6.046239229258517867, -3.283357778048667797 ) ) ;
#1535=VECTOR ( 'NONE', #2073, 1000.000000000000227 ) ;
#1536=CARTESIAN_POINT ( 'NONE',  ( 32.02836186724004364, -4.178063784105134459, -7.939653947423662039 ) ) ;
#1539=CARTESIAN_POINT ( 'NONE',  ( 27.89118264539014547, -6.557423775948280742, -6.861505862736167138 ) ) ;
#1546=CARTESIAN_POINT ( 'NONE',  ( 37.96876116389215383, 4.574485896386907058, 3.995355914169179040E-15 ) ) ;
#1550=CARTESIAN_POINT ( 'NONE',  ( 30.65370992780335868, -5.597623261208691581, -3.627061608673667781 ) ) ;
#1560=DIRECTION ( 'NONE',  ( 0.9928203230275512992, 0.1196152422706610180, 4.006172263299093133E-17 ) ) ;
#1561=CARTESIAN_POINT ( 'NONE',  ( 31.03206908560819954, -5.751910973953721751, -3.283357778048667797 ) ) ;
#1563=CARTESIAN_POINT ( 'NONE',  ( 29.41022140756759029, -3.239556939666760726, -7.939653947423660263 ) ) ;
#1567=FACE_OUTER_BOUND ( 'NONE', #7937, .T. ) ;
#1576=ORIENTED_EDGE ( 'NONE', *, *, #5500, .T. ) ;
#1581=CARTESIAN_POINT ( 'NONE',  ( 32.22908376348204484, -1.973160382215000785, -7.033357778048658027 ) ) ;
#1594=ORIENTED_EDGE ( 'NONE', *, *, #2189, .T. ) ;
#1603=CARTESIAN_POINT ( 'NONE',  ( 32.08959525433819238, -2.916745304588811649, -7.939653947423660263 ) ) ;
#1604=DIRECTION ( 'NONE',  ( -0.1196152422706611984, 0.9928203230275511881, 0.000000000000000000 ) ) ;
#1613=CARTESIAN_POINT ( 'NONE',  ( 31.29094215978502902, -2.813094711071706389, -3.283357778048662023 ) ) ;
#1624=CARTESIAN_POINT ( 'NONE',  ( 28.55903157092087952, -3.142235986053133256, -8.283357778048658915 ) ) ;
#1627=CARTESIAN_POINT ( 'NONE',  ( 30.25533603959949502, -6.272589980291270351, -6.861505862736166250 ) ) ;
#1629=CARTESIAN_POINT ( 'NONE',  ( 25.86833963875586306, -3.039313213345869791, -4.705209693361160461 ) ) ;
#1637=CARTESIAN_POINT ( 'NONE',  ( 33.95908713831676096, -3.945449517755638791, -3.283357778048664688 ) ) ;
#1638=EDGE_CURVE ( 'NONE', #13726, #15016, #7876, .T. ) ;
#1640=CARTESIAN_POINT ( 'NONE',  ( 25.71748644841968456, -2.420320648352046078, -5.783357778048663356 ) ) ;
#1641=CARTESIAN_POINT ( 'NONE',  ( 29.82181869931131146, -4.443908660051686610, -3.627061608673664672 ) ) ;
#1650=DIRECTION ( 'NONE',  ( 0.7752790601682258975, -0.5233950504778124291, -0.3535533905932748411 ) ) ;
#1662=EDGE_CURVE ( 'NONE', #16642, #4757, #14659, .T. ) ;
#1666=DIRECTION ( 'NONE',  ( 0.1196152422706596996, -0.9928203230275514102, 0.000000000000000000 ) ) ;
#1667=CARTESIAN_POINT ( 'NONE',  ( 31.21213704492286212, -2.822589171134389563, -3.283357778048662023 ) ) ;
#1679=ORIENTED_EDGE ( 'NONE', *, *, #11476, .T. ) ;
#1688=CARTESIAN_POINT ( 'NONE',  ( 32.81641299864316608, -4.083119185552795294, -7.939653947423662039 ) ) ;
#1701=VERTEX_POINT ( 'NONE', #13439 ) ;
#1710=CARTESIAN_POINT ( 'NONE',  ( 27.29814976067589072, -3.294147343736873346, -8.283357778048658915 ) ) ;
#1711=CARTESIAN_POINT ( 'NONE',  ( 32.97895737133300287, -1.545456804875373402, -5.113484796970854340 ) ) ;
#1713=CARTESIAN_POINT ( 'NONE',  ( 30.76748005699505129, -4.329975141788874993, -7.939653947423662039 ) ) ;
#1717=CARTESIAN_POINT ( 'NONE',  ( 26.65222088368961195, -7.333664733486695120, -5.783357778048669573 ) ) ;
#1718=CARTESIAN_POINT ( 'NONE',  ( 27.02423718196931546, -4.780961985016209503, -3.283357778048664688 ) ) ;
#1720=ORIENTED_EDGE ( 'NONE', *, *, #10977, .T. ) ;
#1725=DIRECTION ( 'NONE',  ( -0.9928203230275511881, -0.1196152422706606572, -1.761484381769779444E-15 ) ) ;
#1728=CARTESIAN_POINT ( 'NONE',  ( 25.72395281601508898, -4.937620572523835349, -7.939653947423662039 ) ) ;
#1733=UNCERTAINTY_MEASURE_WITH_UNIT (LENGTH_MEASURE( 1.000000000000000082E-05 ), #3980, 'distance_accuracy_value', 'NONE');
#1734=CARTESIAN_POINT ( 'NONE',  ( 27.80031630502317341, -2.169380783275094426, -6.453230759126464378 ) ) ;
#1760=CARTESIAN_POINT ( 'NONE',  ( 31.27600417729400917, -6.449428405189353342, -7.033357778048666908 ) ) ;
#1762=CARTESIAN_POINT ( 'NONE',  ( 29.35089333861488115, -5.954459450865362768, -8.283357778048664244 ) ) ;
#1774=DIRECTION ( 'NONE',  ( -0.1196152422706609625, 0.9928203230275510771, -4.694733121053619507E-17 ) ) ;
#1794=CARTESIAN_POINT ( 'NONE',  ( 26.88845778707760914, -3.543379655034240905, -7.939653947423660263 ) ) ;
#1797=CARTESIAN_POINT ( 'NONE',  ( 31.15208055228630357, -2.102918000029084578, -4.533357778048659803 ) ) ;
#1803=CARTESIAN_POINT ( 'NONE',  ( 47.10521669518294630, -4.378041487036768764, -5.783357778048661579 ) ) ;
#1808=CARTESIAN_POINT ( 'NONE',  ( 33.14902674121363901, -1.535163666906202318, -5.783357778048658027 ) ) ;
#1813=CARTESIAN_POINT ( 'NONE',  ( 30.25080928106424594, -3.138282701210941994, -3.627061608673662896 ) ) ;
#1814=CARTESIAN_POINT ( 'NONE',  ( 26.37178701114681800, -2.351687214456304797, -5.783357778048658915 ) ) ;
#1826=CARTESIAN_POINT ( 'NONE',  ( 26.03917326857634151, -4.899642733102906433, -3.627061608673664672 ) ) ;
#1828=CARTESIAN_POINT ( 'NONE',  ( 26.01652455409633902, -4.902371455920926380, -5.783357778048663356 ) ) ;
#1832=ORIENTED_EDGE ( 'NONE', *, *, #5500, .F. ) ;
#1834=CONICAL_SURFACE ( 'NONE', #7613, 3.425051884552432480, 0.7853981633974544962 ) ;
#1838=DIRECTION ( 'NONE',  ( 0.05980762113533042573, -0.4964101615137759826, 0.8660254037844383745 ) ) ;
#1839=VECTOR ( 'NONE', #13387, 999.9999999999998863 ) ;
#1857=CARTESIAN_POINT ( 'NONE',  ( 28.48706592061337162, -2.086641016831144668, -5.113484796970857893 ) ) ;
#1859=CARTESIAN_POINT ( 'NONE',  ( 31.03206908560819954, -5.751910973953720863, -3.283357778048667797 ) ) ;
#1860=CARTESIAN_POINT ( 'NONE',  ( 29.37220822929407760, -7.016156836349003001, -5.783357778048668685 ) ) ;
#1868=FACE_OUTER_BOUND ( 'NONE', #16030, .T. ) ;
#1874=LINE ( 'NONE', #7403, #10487 ) ;
#1881=CARTESIAN_POINT ( 'NONE',  ( 32.93018312783485158, -2.815471066132994249, -3.627061608673662008 ) ) ;
#1882=FACE_OUTER_BOUND ( 'NONE', #9076, .T. ) ;
#1889=CARTESIAN_POINT ( 'NONE',  ( 32.57506351453486815, -6.630276025878011126, -5.113484796970860558 ) ) ;
#1893=PLANE ( 'NONE',  #6940 ) ;
#1896=CARTESIAN_POINT ( 'NONE',  ( 26.15738093914773543, -4.885401043216321959, -8.283357778048662468 ) ) ;
#1898=CARTESIAN_POINT ( 'NONE',  ( 38.70301816123731697, -5.700001250565210675, -9.783357778048662468 ) ) ;
#1901=CARTESIAN_POINT ( 'NONE',  ( 27.61527553138257574, -4.709753535998224550, -7.939653947423662039 ) ) ;
#1902=EDGE_LOOP ( 'NONE', ( #17507, #1500, #6103, #12503 ) ) ;
#1905=ADVANCED_FACE ( 'NONE', ( #5430 ), #6623, .T. ) ;
#1911=CARTESIAN_POINT ( 'NONE',  ( 33.76207435632690590, -3.969185667289998332, -3.627061608673664672 ) ) ;
#1913=EDGE_CURVE ( 'NONE', #16642, #16315, #12251, .T. ) ;
#1915=CARTESIAN_POINT ( 'NONE',  ( 25.77727992838053339, -5.625024813964539128, -7.939653947423662927 ) ) ;
#1924=ORIENTED_EDGE ( 'NONE', *, *, #8512, .F. ) ;
#1933=EDGE_LOOP ( 'NONE', ( #3187, #9440 ) ) ;
#1934=CYLINDRICAL_SURFACE ( 'NONE', #7061, 2.500000000000001776 ) ;
#1935=EDGE_LOOP ( 'NONE', ( #10375, #16501, #8325, #11917 ) ) ;
#1945=CARTESIAN_POINT ( 'NONE',  ( 31.84257795004535652, -2.746633492292519296, -3.283357778048662023 ) ) ;
#1946=EDGE_CURVE ( 'NONE', #627, #82, #13487, .T. ) ;
#1947=CYLINDRICAL_SURFACE ( 'NONE', #2819, 2.500000000000001776 ) ;
#1951=CARTESIAN_POINT ( 'NONE',  ( 30.41656616297672500, -2.191532958677927745, -7.033357778048658027 ) ) ;
#1967=ORIENTED_EDGE ( 'NONE', *, *, #1296, .F. ) ;
#1969=ADVANCED_FACE ( 'NONE', ( #7261 ), #10140, .T. ) ;
#1972=ORIENTED_EDGE ( 'NONE', *, *, #14626, .F. ) ;
#1974=CARTESIAN_POINT ( 'NONE',  ( 31.88017671309158274, -6.376637546091784792, -4.533357778048668685 ) ) ;
#1981=CARTESIAN_POINT ( 'NONE',  ( 27.10304229683147526, -4.771467524953526329, -3.283357778048664688 ) ) ;
#1985=CARTESIAN_POINT ( 'NONE',  ( 27.10313151398701947, -6.652368374500619908, -6.861505862736166250 ) ) ;
#1986=CARTESIAN_POINT ( 'NONE',  ( 25.76775864925888015, -2.837585720338237749, -6.439571894700457655 ) ) ;
#1997=LINE ( 'NONE', #3348, #3999 ) ;
#2000=CARTESIAN_POINT ( 'NONE',  ( 32.50119254608192421, -4.121097024973739309, -3.627061608673664672 ) ) ;
#2001=CARTESIAN_POINT ( 'NONE',  ( 30.37154917142620292, -2.923863409590206519, -8.283357778048660691 ) ) ;
#2023=CARTESIAN_POINT ( 'NONE',  ( 28.74176732417158320, -7.092112515190875044, -5.783357778048657138 ) ) ;
#2031=DIRECTION ( 'NONE',  ( 0.9928203230275510771, 0.1196152422706609902, 4.006172263299092517E-17 ) ) ;
#2032=CARTESIAN_POINT ( 'NONE',  ( 28.51030546511822195, -6.055733689321201041, -3.283357778048667797 ) ) ;
#2034=LINE ( 'NONE', #3299, #16713 ) ;
#2039=CARTESIAN_POINT ( 'NONE',  ( 30.71189515440122975, -6.854751018602581958, -5.783357778048663356 ) ) ;
#2044=CARTESIAN_POINT ( 'NONE',  ( 25.81704846941310549, -3.246696919197674447, -4.409389677717624245 ) ) ;
#2047=ORIENTED_EDGE ( 'NONE', *, *, #16346, .F. ) ;
#2055=ORIENTED_EDGE ( 'NONE', *, *, #15818, .F. ) ;
#2057=CARTESIAN_POINT ( 'NONE',  ( 30.19827253897071273, -3.144612341114420673, -7.939653947423660263 ) ) ;
#2064=CARTESIAN_POINT ( 'NONE',  ( 26.66961417369883591, -4.823687054261037055, -3.627061608673664672 ) ) ;
#2069=CIRCLE ( 'NONE', #1483, 2.499999999999999556 ) ;
#2073=DIRECTION ( 'NONE',  ( 0.9928203230275510771, 0.1196152422706609902, 4.006172263299092517E-17 ) ) ;
#2075=CARTESIAN_POINT ( 'NONE',  ( 27.41826274939272423, -4.733489685532582314, -8.283357778048662468 ) ) ;
#2078=LINE ( 'NONE', #13396, #17368 ) ;
#2080=CARTESIAN_POINT ( 'NONE',  ( 26.66961417369883591, -4.823687054261037055, -3.627061608673664672 ) ) ;
#2093=CARTESIAN_POINT ( 'NONE',  ( 29.45101334415624095, -7.006662376286321603, -5.783357778048657138 ) ) ;
#2095=CARTESIAN_POINT ( 'NONE',  ( 33.35047706458318828, -2.764833946905071560, -7.939653947423660263 ) ) ;
#2107=CARTESIAN_POINT ( 'NONE',  ( 32.08959525433819238, -2.916745304588811205, -7.939653947423660263 ) ) ;
#2117=AXIS2_PLACEMENT_3D ( 'NONE', #17022, #2859, #1604 ) ;
#2118=AXIS2_PLACEMENT_3D ( 'NONE', #9262, #13257, #7651 ) ;
#2119=CARTESIAN_POINT ( 'NONE',  ( 29.54600080245929306, -4.477139269648729325, -3.283357778048664688 ) ) ;
#2120=CARTESIAN_POINT ( 'NONE',  ( 28.51030546511822195, -6.055733689321201041, -3.283357778048667797 ) ) ;
#2123=CARTESIAN_POINT ( 'NONE',  ( 29.98133424373737199, -5.878503772023492502, -8.283357778048664244 ) ) ;
#2131=CARTESIAN_POINT ( 'NONE',  ( 29.11066736118121057, -3.075774767273946608, -8.283357778048658915 ) ) ;
#2143=CARTESIAN_POINT ( 'NONE',  ( 25.80685721358263152, -3.162108319002908896, -4.519686641326834398 ) ) ;
#2150=FACE_OUTER_BOUND ( 'NONE', #10317, .T. ) ;
#2151=CARTESIAN_POINT ( 'NONE',  ( 30.17635249042624679, -2.520282741259753045, -6.861505862736158257 ) ) ;
#2153=DIRECTION ( 'NONE',  ( -0.1196152422706609625, 0.9928203230275510771, 0.000000000000000000 ) ) ;
#2157=EDGE_CURVE ( 'NONE', #692, #13923, #12313, .T. ) ;
#2159=CARTESIAN_POINT ( 'NONE',  ( 26.98483462626008134, -4.785709214840094816, -7.939653947423662039 ) ) ;
#2163=CARTESIAN_POINT ( 'NONE',  ( 27.50903986916043920, -7.240631829073577386, -6.453230759126468818 ) ) ;
#2166=CARTESIAN_POINT ( 'NONE',  ( 25.95642634701329499, -4.403549397486667516, -3.686412874245489135 ) ) ;
#2171=CARTESIAN_POINT ( 'NONE',  ( 32.56242593318007295, -2.859778545457410281, -7.939653947423660263 ) ) ;
#2174=CARTESIAN_POINT ( 'NONE',  ( 27.72904566057427189, -3.442105416578422172, -3.627061608673662896 ) ) ;
#2187=CARTESIAN_POINT ( 'NONE',  ( 29.66420847303068697, -4.462897579762144851, -7.939653947423662039 ) ) ;
#2189=EDGE_CURVE ( 'NONE', #3360, #2203, #14783, .T. ) ;
#2191=CARTESIAN_POINT ( 'NONE',  ( 33.00219691583784964, -5.514549477365426888, -3.283357778048667797 ) ) ;
#2198=CARTESIAN_POINT ( 'NONE',  ( 31.44176105920648112, -5.502678662656354192, -3.627061608673668225 ) ) ;
#2202=EDGE_CURVE ( 'NONE', #9429, #14403, #16502, .T. ) ;
#2203=VERTEX_POINT ( 'NONE', #17344 ) ;
#2215=CARTESIAN_POINT ( 'NONE',  ( 26.11428532722776197, -5.713797161519015511, -3.668609639089262409 ) ) ;
#2218=CARTESIAN_POINT ( 'NONE',  ( 29.41846958523816724, -7.400131432564565515, -5.783357778048669573 ) ) ;
#2219=CARTESIAN_POINT ( 'NONE',  ( 31.88814493096864311, -1.687075024589942407, -5.783357778048658915 ) ) ;
#2223=CARTESIAN_POINT ( 'NONE',  ( 26.64639396487419987, -2.308405637095112706, -5.783357778048658027 ) ) ;
#2228=CARTESIAN_POINT ( 'NONE',  ( 25.89388370423996832, -3.884438240559767053, -3.881334880282079514 ) ) ;
#2237=CARTESIAN_POINT ( 'NONE',  ( 31.44176105920648823, -5.502678662656354192, -3.627061608673668225 ) ) ;
#2239=CARTESIAN_POINT ( 'NONE',  ( 26.07857582428556853, -4.894895503279006022, -8.283357778048662468 ) ) ;
#2241=ORIENTED_EDGE ( 'NONE', *, *, #2202, .T. ) ;
#2243=ORIENTED_EDGE ( 'NONE', *, *, #6742, .F. ) ;
#2252=CARTESIAN_POINT ( 'NONE',  ( 32.51858583609114106, -1.611119345748072362, -5.783357778048658027 ) ) ;
#2255=CARTESIAN_POINT ( 'NONE',  ( 31.95146207396702565, -5.641142275435199416, -8.283357778048664244 ) ) ;
#2256=CARTESIAN_POINT ( 'NONE',  ( 27.62849893492243325, -6.589071975465733644, -4.705209693361168455 ) ) ;
#2269=( BOUNDED_CURVE ( )  B_SPLINE_CURVE ( 2, ( #214, #5722, #11240, #16816, #4817, #7292, #5816, #11525, #10259 ),
 .UNSPECIFIED., .F., .T. ) 
 B_SPLINE_CURVE_WITH_KNOTS ( ( 3, 2, 2, 2, 3 ),
 ( 0.2500000000000000000, 0.2564102564102563875, 0.2692307692307692180, 0.2820512820512820484, 0.2884615384615384914 ),
 .UNSPECIFIED. ) 
 CURVE ( )  GEOMETRIC_REPRESENTATION_ITEM ( )  RATIONAL_B_SPLINE_CURVE ( ( 0.9330127018922194093, 0.9330127018922195203, 1.000000000000000000, 0.8660254037844387076, 1.000000000000000000, 0.8660254037844387076, 1.000000000000000000, 0.9330127018922190762, 0.9330127018922194093 ) ) 
 REPRESENTATION_ITEM ( '' )  );
#2270=AXIS2_PLACEMENT_3D ( 'NONE', #16996, #14080, #1666 ) ;
#2273=CARTESIAN_POINT ( 'NONE',  ( 29.52399153675929355, -1.971908820246954130, -5.783357778048658027 ) ) ;
#2276=CARTESIAN_POINT ( 'NONE',  ( 32.41296236253129592, -1.951006642345344044, -4.533357778048659803 ) ) ;
#2278=CARTESIAN_POINT ( 'NONE',  ( 46.70046462172870605, -5.135117178011730843, -5.783357778048661579 ) ) ;
#2282=CARTESIAN_POINT ( 'NONE',  ( 30.92509028327567933, -4.310986222078405206, -7.939653947423662039 ) ) ;
#2288=ORIENTED_EDGE ( 'NONE', *, *, #17671, .F. ) ;
#2289=CARTESIAN_POINT ( 'NONE',  ( 33.14105852333657509, -6.224726188408045147, -4.533357778048668685 ) ) ;
#2294=CARTESIAN_POINT ( 'NONE',  ( 27.82847066025702887, -2.165988739474055791, -5.783357778048658027 ) ) ;
#2296=B_SPLINE_CURVE_WITH_KNOTS ( 'NONE', 1,
 ( #16667, #17795 ),
 .UNSPECIFIED., .F., .F.,
 ( 2, 2 ),
 ( 0.000000000000000000, 1.000000000000000000 ),
 .UNSPECIFIED. ) ;
#2303=CARTESIAN_POINT ( 'NONE',  ( 25.71748644841968456, -2.420320648352046078, -5.783357778048663356 ) ) ;
#2306=CARTESIAN_POINT ( 'NONE',  ( 27.33945763453056088, -4.742984145595265488, -8.283357778048662468 ) ) ;
#2307=CARTESIAN_POINT ( 'NONE',  ( 31.51169109130924184, -2.986371343527201905, -3.627061608673662896 ) ) ;
#2328=CARTESIAN_POINT ( 'NONE',  ( 30.82871344409320713, -3.068656662272551738, -7.939653947423660263 ) ) ;
#2332=CIRCLE ( 'NONE', #11565, 3.000000000000001332 ) ;
#2345=CARTESIAN_POINT ( 'NONE',  ( 31.49429780130001433, -5.496349022752856861, -7.939653947423664704 ) ) ;
#2357=EDGE_LOOP ( 'NONE', ( #15581, #5028, #8207, #8002 ) ) ;
#2367=CARTESIAN_POINT ( 'NONE',  ( 30.17635249042624679, -2.520282741259753045, -6.861505862736158257 ) ) ;
#2369=CARTESIAN_POINT ( 'NONE',  ( 32.97211790677835097, -2.610546234160043610, -8.283357778048658915 ) ) ;
#2370=CARTESIAN_POINT ( 'NONE',  ( 27.55969062878875064, -7.234529412811931515, -5.783357778048668685 ) ) ;
#2376=CARTESIAN_POINT ( 'NONE',  ( 31.65190802758064592, -5.477360103042387074, -7.939653947423662927 ) ) ;
#2381=ORIENTED_EDGE ( 'NONE', *, *, #14225, .F. ) ;
#2397=PLANE ( 'NONE',  #15592 ) ;
#2398=CARTESIAN_POINT ( 'NONE',  ( 33.30246708102489350, -5.905470865888903020, -4.705209693361168455 ) ) ;
#2401=ADVANCED_FACE ( 'NONE', ( #16331 ), #14949, .T. ) ;
#2407=PLANE ( 'NONE',  #4145 ) ;
#2408=EDGE_CURVE ( 'NONE', #16712, #14075, #6866, .T. ) ;
#2412=CARTESIAN_POINT ( 'NONE',  ( 26.18940075748478691, -6.337263906362392341, -7.823530922983556124 ) ) ;
#2413=CARTESIAN_POINT ( 'NONE',  ( 29.34898802046944155, -4.500875419183088866, -3.627061608673664672 ) ) ;
#2416=ORIENTED_EDGE ( 'NONE', *, *, #6251, .T. ) ;
#2417=ADVANCED_FACE ( 'NONE', ( #17882 ), #1174, .T. ) ;
#2422=CARTESIAN_POINT ( 'NONE',  ( 33.15485366002904755, -6.560422763297783177, -5.783357778048663356 ) ) ;
#2433=ORIENTED_EDGE ( 'NONE', *, *, #10552, .F. ) ;
#2436=CARTESIAN_POINT ( 'NONE',  ( 33.06225340847440464, -6.234220648470727433, -4.533357778048668685 ) ) ;
#2441=EDGE_LOOP ( 'NONE', ( #11394, #4885, #245, #3297 ) ) ;
#2445=CARTESIAN_POINT ( 'NONE',  ( 31.26353094466156080, -6.788289799823394866, -5.783357778048663356 ) ) ;
#2446=CARTESIAN_POINT ( 'NONE',  ( 29.78612525785423060, -2.267488637519798012, -7.033357778048658027 ) ) ;
#2448=CARTESIAN_POINT ( 'NONE',  ( 28.28955653359400557, -5.882457056865704637, -3.627061608673668225 ) ) ;
#2451=CARTESIAN_POINT ( 'NONE',  ( 33.14105852333657509, -6.224726188408045147, -4.533357778048668685 ) ) ;
#2456=EDGE_CURVE ( 'NONE', #6239, #17548, #9643, .T. ) ;
#2458=CARTESIAN_POINT ( 'NONE',  ( 33.54323074294813267, -5.249493066516778050, -7.939653947423662927 ) ) ;
#2467=CARTESIAN_POINT ( 'NONE',  ( 26.01595305975170547, -2.384361315936983416, -5.783357778048670461 ) ) ;
#2476=CARTESIAN_POINT ( 'NONE',  ( 26.30185955129047315, -7.986322017489088765, -6.648778972250404706 ) ) ;
#2477=CARTESIAN_POINT ( 'NONE',  ( 32.67202617590239555, -5.981426544730773287, -4.705209693361168455 ) ) ;
#2478=EDGE_CURVE ( 'NONE', #6885, #5290, #17097, .T. ) ;
#2479=CARTESIAN_POINT ( 'NONE',  ( 32.30788887834420819, -1.963665922152317833, -7.033357778048658027 ) ) ;
#2489=CARTESIAN_POINT ( 'NONE',  ( 33.48996557372703364, -1.821249024531260696, -7.033357778048658027 ) ) ;
#2499=CARTESIAN_POINT ( 'NONE',  ( 27.87986455999572399, -6.131689368163070419, -3.283357778048667797 ) ) ;
#2500=VERTEX_POINT ( 'NONE', #3463 ) ;
#2520=ORIENTED_EDGE ( 'NONE', *, *, #1638, .F. ) ;
#2523=CARTESIAN_POINT ( 'NONE',  ( 28.39010325924584421, -2.735490497978389612, -4.705209693361160461 ) ) ;
#2525=CARTESIAN_POINT ( 'NONE',  ( 32.14656953781143756, -4.163822094218565972, -3.283357778048664688 ) ) ;
#2526=CARTESIAN_POINT ( 'NONE',  ( 26.01652455409633902, -4.902371455920926380, -5.783357778048663356 ) ) ;
#2530=PRESENTATION_STYLE_ASSIGNMENT (( #15260 ) ) ;
#2533=CARTESIAN_POINT ( 'NONE',  ( 28.26310972651430120, -2.123820177930694442, -5.783357778048658915 ) ) ;
#2538=EDGE_CURVE ( 'NONE', #9123, #16897, #3649, .T. ) ;
#2539=EDGE_CURVE ( 'NONE', #6798, #6479, #11500, .T. ) ;
#2560=CARTESIAN_POINT ( 'NONE',  ( 33.40301380667672504, -2.758504307001591993, -3.627061608673662896 ) ) ;
#2562=CARTESIAN_POINT ( 'NONE',  ( 32.61569110240115776, -6.288022587442930522, -7.033357778048666908 ) ) ;
#2574=LINE ( 'NONE', #8461, #13241 ) ;
#2575=CARTESIAN_POINT ( 'NONE',  ( 33.76397967447234549, -5.422769698972272678, -8.283357778048662468 ) ) ;
#2585=ORIENTED_EDGE ( 'NONE', *, *, #15391, .F. ) ;
#2588=CARTESIAN_POINT ( 'NONE',  ( 34.25812524399339765, -6.427500325324518649, -5.783357778048663356 ) ) ;
#2593=DIRECTION ( 'NONE',  ( -0.9928203230275510771, -0.1196152422706614760, -0.000000000000000000 ) ) ;
#2599=DIRECTION ( 'NONE',  ( -0.1196152422706610735, 0.9928203230275511881, 0.000000000000000000 ) ) ;
#2600=CARTESIAN_POINT ( 'NONE',  ( 38.42250453410443356, 0.8083635290851024502, -5.533357778048658027 ) ) ;
#2601=ORIENTED_EDGE ( 'NONE', *, *, #7106, .T. ) ;
#2616=CARTESIAN_POINT ( 'NONE',  ( 26.60838078660069428, -6.085005533777348319, -7.939653947423664704 ) ) ;
#2618=CARTESIAN_POINT ( 'NONE',  ( 29.21955148510287614, -5.970283550416647600, -3.283357778048667797 ) ) ;
#2628=CARTESIAN_POINT ( 'NONE',  ( 27.63266882139180325, -2.199775856772564708, -5.783357778048658915 ) ) ;
#2629=VECTOR ( 'NONE', #10486, 1000.000000000000227 ) ;
#2639=CARTESIAN_POINT ( 'NONE',  ( 28.13194630731337753, -5.901445976576171759, -3.627061608673667781 ) ) ;
#2640=DIRECTION ( 'NONE',  ( 0.9928203230275510771, 0.1196152422706609902, 4.006172263299092517E-17 ) ) ;
#2649=DIRECTION ( 'NONE',  ( -0.1196152422706610735, 0.9928203230275511881, 0.000000000000000000 ) ) ;
#2650=LINE ( 'NONE', #12157, #17653 ) ;
#2651=SHAPE_REPRESENTATION ( 'Bleed Screw Nipple', ( #3575 ), #12173 ) ;
#2652=CARTESIAN_POINT ( 'NONE',  ( 29.50659824675005893, -4.481886499472614638, -7.939653947423662039 ) ) ;
#2656=EDGE_CURVE ( 'NONE', #757, #9716, #17174, .T. ) ;
#2657=VERTEX_POINT ( 'NONE', #6548 ) ;
#2668=CARTESIAN_POINT ( 'NONE',  ( 25.93488947238681774, -5.606027099510431988, -7.939653947423663816 ) ) ;
#2676=AXIS2_PLACEMENT_3D ( 'NONE', #16925, #5738, #17108 ) ;
#2679=ORIENTED_EDGE ( 'NONE', *, *, #340, .F. ) ;
#2692=CARTESIAN_POINT ( 'NONE',  ( 25.71748644841968456, -2.420320648352046078, -5.783357778048663356 ) ) ;
#2694=AXIS2_PLACEMENT_3D ( 'NONE', #17204, #949, #3586 ) ;
#2697=ADVANCED_FACE ( 'NONE', ( #10867 ), #8084, .T. ) ;
#2700=DIRECTION ( 'NONE',  ( 0.9928203230275512992, 0.1196152422706610180, 4.006172263299093133E-17 ) ) ;
#2702=VERTEX_POINT ( 'NONE', #8345 ) ;
#2708=CARTESIAN_POINT ( 'NONE',  ( 26.37178701114681800, -2.351687214456304353, -5.783357778048658027 ) ) ;
#2710=ORIENTED_EDGE ( 'NONE', *, *, #2456, .T. ) ;
#2711=CARTESIAN_POINT ( 'NONE',  ( 29.89119874204131122, -2.254829357712824667, -4.533357778048659803 ) ) ;
#2713=CARTESIAN_POINT ( 'NONE',  ( 32.60321786976872005, -6.626883982076972046, -5.783357778048663356 ) ) ;
#2716=ORIENTED_EDGE ( 'NONE', *, *, #10180, .F. ) ;
#2719=CARTESIAN_POINT ( 'NONE',  ( 30.19827253897071273, -3.144612341114421561, -7.939653947423660263 ) ) ;
#2730=CARTESIAN_POINT ( 'NONE',  ( 28.73594040535616756, -2.066853418799292630, -5.783357778048658027 ) ) ;
#2743=CARTESIAN_POINT ( 'NONE',  ( 28.36401332423200827, -6.500457016816879374, -6.861505862736166250 ) ) ;
#2757=CARTESIAN_POINT ( 'NONE',  ( 27.75966235412334981, -2.811446176820259879, -4.705209693361160461 ) ) ;
#2759=ORIENTED_EDGE ( 'NONE', *, *, #9974, .T. ) ;
#2767=VERTEX_POINT ( 'NONE', #15327 ) ;
#2770=ORIENTED_EDGE ( 'NONE', *, *, #14348, .F. ) ;
#2774=CARTESIAN_POINT ( 'NONE',  ( 28.36392410707646761, -4.619556167269785796, -3.283357778048664688 ) ) ;
#2783=CARTESIAN_POINT ( 'NONE',  ( 28.53771668024168662, -2.080538600569502794, -5.783357778048658027 ) ) ;
#2790=CARTESIAN_POINT ( 'NONE',  ( 26.85044460880409645, -7.319979551716484067, -5.783357778048668685 ) ) ;
#2791=CARTESIAN_POINT ( 'NONE',  ( 28.52524344760924180, -2.419399995203538101, -7.033357778048658027 ) ) ;
#2796=CARTESIAN_POINT ( 'NONE',  ( 28.39010325924584421, -2.735490497978389612, -4.705209693361160461 ) ) ;
#2801=EDGE_LOOP ( 'NONE', ( #3087, #14366, #10262, #4581, #2416, #1972 ) ) ;
#2805=CARTESIAN_POINT ( 'NONE',  ( 32.21340264088064487, -1.637691031382005669, -6.453230759126468818 ) ) ;
#2808=CARTESIAN_POINT ( 'NONE',  ( 28.14933959732260149, -3.391468297350501260, -7.939653947423660263 ) ) ;
#2809=CARTESIAN_POINT ( 'NONE',  ( 28.43075721014566781, -2.093425104433228157, -6.453230759126469707 ) ) ;
#2811=DIRECTION ( 'NONE',  ( -0.1196152422706610735, 0.9928203230275511881, 0.000000000000000000 ) ) ;
#2818=CARTESIAN_POINT ( 'NONE',  ( 31.17093069310692499, -6.462087684996337345, -4.533357778048668685 ) ) ;
#2819=AXIS2_PLACEMENT_3D ( 'NONE', #9984, #10346, #6188 ) ;
#2820=CARTESIAN_POINT ( 'NONE',  ( 28.56093688906631911, -4.595820017735426255, -3.627061608673664672 ) ) ;
#2824=ORIENTED_EDGE ( 'NONE', *, *, #13327, .F. ) ;
#2834=AXIS2_PLACEMENT_3D ( 'NONE', #16697, #7184, #7369 ) ;
#2835=CARTESIAN_POINT ( 'NONE',  ( 28.52162355051263987, -6.481468097106410475, -6.861505862736167138 ) ) ;
#2846=ORIENTED_EDGE ( 'NONE', *, *, #17557, .T. ) ;
#2847=CARTESIAN_POINT ( 'NONE',  ( 27.29063000668916672, -2.568146533142987575, -4.533357778048659803 ) ) ;
#2849=( BOUNDED_SURFACE ( )  B_SPLINE_SURFACE ( 1, 2, ( 
 ( #11911, #9285, #14827, #17586, #13375, #957, #7848, #16199, #5106, #3764, #10626, #12005, #6490, #260, #11285, #7070, #2984, #11387, #8785, #11191, #16862, #9938, #13942, #4511, #9750, #448, #10027, #7157, #4426, #12861, #1536, #16955, #15575, #5950, #11474, #17042, #15488, #4249, #12587, #10118, #12667, #166, #3070, #4333, #15302, #15669, #5770, #8590, #5677, #8505, #3154, #14318, #16762, #14125, #1713, #9845, #8690, #2883, #4597, #14219, #7245, #1813, #15397, #7342, #3249, #14040, #6964, #12494, #1627, #12761, #8410, #356, #5864, #81, #5590, #16675, #11107, #9137, #13129, #10216, #5044, #11843, #14495, #4775, #6142, #620, #4689, #9046, #10566, #15765, #13217, #16130, #17236, #16046, #3338, #11752, #11934, #4952, #793, #6321, #14599, #17420, #11571, #3692, #10298, #6416, #10481, #15944, #707, #2174, #9217, #17321, #11668, #3614, #1901, #15849, #527, #14675, #2256, #8869, #7773, #13302, #884, #14402, #17523, #3423, #7426, #12941, #1985, #7689, #6042, #17139, #2080, #7508, #13031, #4862, #8954, #7603, #6232, #3514, #10391, #10229, #8969, #7526, #1826, #7358, #14332, #8800, #15777, #6157, #1728, #1915, #5879 ),
 ( #3084, #14512, #632, #4612, #7258, #2095, #3351, #5963, #14237, #15589, #10041, #14138, #541, #7619, #12776, #4702, #13142, #8705, #13047, #372, #3265, #3439, #14418, #8884, #2000, #6056, #11681, #8606, #721, #12875, #15867, #17251, #7437, #10136, #11585, #11300, #12957, #3166, #4790, #16879, #460, #9952, #10310, #4441, #11403, #15503, #16967, #4524, #11489, #17058, #15684, #17153, #17623, #9062, #998, #13588, #1076, #6433, #13228, #6599, #16146, #15963, #10499, #11860, #2367, #3889, #9230, #901, #13503, #14860, #11956, #3707, #6523, #5229, #14609, #2273, #17439, #12129, #2187, #14779, #17538, #7884, #17709, #806, #16232, #3805, #10751, #16327, #9404, #10579, #3530, #6336, #14946, #5058, #4970, #13417, #3630, #7702, #2523, #12035, #5142, #16060, #7791, #10660, #8050, #9152, #9321, #2448, #14691, #7971, #13321, #6246, #11767, #17340, #4878, #10408, #16669, #5672, #15121, #11183, #7060, #4059, #6954, #15028, #5492, #16756, #12486, #15208, #17960, #8312, #4327, #16575, #17879, #5584, #2976, #2708, #17798, #4241, #13935, #2616, #11101, #1530, #160, #13675, #15295, #5402, #72, #9741, #3974, #13844, #8499, #12579, #1341 ) ),
 .UNSPECIFIED., .F., .F., .T. ) 
 B_SPLINE_SURFACE_WITH_KNOTS ( ( 2, 2 ),
 ( 3, 2, 2, 2, 2, 2, 2, 2, 2, 2, 2, 2, 2, 2, 2, 2, 2, 2, 2, 2, 2, 2, 2, 2, 2, 2, 2, 2, 2, 2, 2, 2, 2, 2, 2, 2, 2, 2, 2, 2, 2, 2, 2, 2, 2, 2, 2, 2, 2, 2, 2, 2, 2, 2, 2, 2, 2, 2, 2, 2, 2, 2, 2, 2, 2, 2, 2, 2, 2, 2, 2, 2, 2, 2, 2, 2, 3 ),
 ( 0.000000000000000000, 1.000000000000000000 ),
 ( 0.000000000000000000, 0.01282051282051282007, 0.02564102564102564014, 0.03846153846153846367, 0.05128205128205128027, 0.06410256410256409687, 0.07692307692307692735, 0.08974358974358974395, 0.1025641025641025605, 0.1153846153846153910, 0.1282051282051281937, 0.1410256410256410242, 0.1538461538461538547, 0.1666666666666666574, 0.1794871794871794879, 0.1923076923076923184, 0.2051282051282051211, 0.2179487179487179516, 0.2307692307692307820, 0.2435897435897435848, 0.2564102564102563875, 0.2692307692307692180, 0.2820512820512820484, 0.2948717948717948789, 0.3076923076923077094, 0.3205128205128205399, 0.3333333333333333148, 0.3461538461538461453, 0.3589743589743589758, 0.3717948717948718063, 0.3846153846153846367, 0.3974358974358974117, 0.4102564102564102422, 0.4230769230769230727, 0.4358974358974359031, 0.4487179487179487336, 0.4615384615384615641, 0.4743589743589743390, 0.4871794871794871695, 0.5000000000000000000, 0.5128205128205127750, 0.5256410256410256610, 0.5384615384615384359, 0.5512820512820513219, 0.5641025641025640969, 0.5769230769230768718, 0.5897435897435897578, 0.6025641025641025328, 0.6153846153846154188, 0.6282051282051281937, 0.6410256410256410797, 0.6538461538461538547, 0.6666666666666666297, 0.6794871794871795156, 0.6923076923076922906, 0.7051282051282051766, 0.7179487179487179516, 0.7307692307692307265, 0.7435897435897436125, 0.7564102564102563875, 0.7692307692307692735, 0.7820512820512820484, 0.7948717948717948234, 0.8076923076923077094, 0.8205128205128204844, 0.8333333333333333703, 0.8461538461538461453, 0.8589743589743589203, 0.8717948717948718063, 0.8846153846153845812, 0.8974358974358974672, 0.9102564102564102422, 0.9230769230769231282, 0.9358974358974359031, 0.9487179487179486781, 0.9615384615384615641, 0.9690838366659333403 ),
 .UNSPECIFIED. ) 
 GEOMETRIC_REPRESENTATION_ITEM ( )  RATIONAL_B_SPLINE_SURFACE ( (
 ( 1.000000000000000000, 0.8660254037844387076, 1.000000000000000000, 0.8660254037844387076, 1.000000000000000000, 0.8660254037844387076, 1.000000000000000000, 0.8660254037844387076, 1.000000000000000000, 0.8660254037844387076, 1.000000000000000000, 0.8660254037844387076, 1.000000000000000000, 0.8660254037844387076, 1.000000000000000000, 0.8660254037844387076, 1.000000000000000000, 0.8660254037844387076, 1.000000000000000000, 0.8660254037844387076, 1.000000000000000000, 0.8660254037844387076, 1.000000000000000000, 0.8660254037844387076, 1.000000000000000000, 0.8660254037844387076, 1.000000000000000000, 0.8660254037844387076, 1.000000000000000000, 0.8660254037844387076, 1.000000000000000000, 0.8660254037844387076, 1.000000000000000000, 0.8660254037844387076, 1.000000000000000000, 0.8660254037844387076, 1.000000000000000000, 0.8660254037844387076, 1.000000000000000000, 0.8660254037844387076, 1.000000000000000000, 0.8660254037844387076, 1.000000000000000000, 0.8660254037844387076, 1.000000000000000000, 0.8660254037844387076, 1.000000000000000000, 0.8660254037844387076, 1.000000000000000000, 0.8660254037844387076, 1.000000000000000000, 0.8660254037844387076, 1.000000000000000000, 0.8660254037844387076, 1.000000000000000000, 0.8660254037844387076, 1.000000000000000000, 0.8660254037844387076, 1.000000000000000000, 0.8660254037844387076, 1.000000000000000000, 0.8660254037844387076, 1.000000000000000000, 0.8660254037844387076, 1.000000000000000000, 0.8660254037844387076, 1.000000000000000000, 0.8660254037844387076, 1.000000000000000000, 0.8660254037844387076, 1.000000000000000000, 0.8660254037844387076, 1.000000000000000000, 0.8660254037844387076, 1.000000000000000000, 0.8660254037844387076, 1.000000000000000000, 0.8660254037844387076, 1.000000000000000000, 0.8660254037844387076, 1.000000000000000000, 0.8660254037844387076, 1.000000000000000000, 0.8660254037844387076, 1.000000000000000000, 0.8660254037844387076, 1.000000000000000000, 0.8660254037844387076, 1.000000000000000000, 0.8660254037844387076, 1.000000000000000000, 0.8660254037844387076, 1.000000000000000000, 0.8660254037844387076, 1.000000000000000000, 0.8660254037844387076, 1.000000000000000000, 0.8660254037844387076, 1.000000000000000000, 0.8660254037844387076, 1.000000000000000000, 0.8660254037844387076, 1.000000000000000000, 0.8660254037844387076, 1.000000000000000000, 0.8660254037844387076, 1.000000000000000000, 0.8660254037844387076, 1.000000000000000000, 0.8660254037844387076, 1.000000000000000000, 0.8660254037844387076, 1.000000000000000000, 0.8660254037844387076, 1.000000000000000000, 0.8660254037844387076, 1.000000000000000000, 0.8660254037844387076, 1.000000000000000000, 0.8660254037844387076, 1.000000000000000000, 0.8660254037844387076, 1.000000000000000000, 0.8660254037844387076, 1.000000000000000000, 0.8660254037844387076, 1.000000000000000000, 0.8660254037844387076, 1.000000000000000000, 0.8660254037844387076, 1.000000000000000000, 0.8660254037844387076, 1.000000000000000000, 0.8660254037844387076, 1.000000000000000000, 0.8660254037844387076, 1.000000000000000000, 0.8660254037844387076, 1.000000000000000000, 0.8660254037844387076, 1.000000000000000000, 0.8660254037844387076, 1.000000000000000000, 0.8660254037844387076, 1.000000000000000000, 0.8660254037844387076, 1.000000000000000000, 0.8660254037844387076, 1.000000000000000000, 0.8660254037844387076, 1.000000000000000000, 0.9211506902921580142, 0.9351132093492240394),
 ( 1.000000000000000000, 0.8660254037844387076, 1.000000000000000000, 0.8660254037844387076, 1.000000000000000000, 0.8660254037844387076, 1.000000000000000000, 0.8660254037844387076, 1.000000000000000000, 0.8660254037844387076, 1.000000000000000000, 0.8660254037844387076, 1.000000000000000000, 0.8660254037844387076, 1.000000000000000000, 0.8660254037844387076, 1.000000000000000000, 0.8660254037844387076, 1.000000000000000000, 0.8660254037844387076, 1.000000000000000000, 0.8660254037844387076, 1.000000000000000000, 0.8660254037844387076, 1.000000000000000000, 0.8660254037844387076, 1.000000000000000000, 0.8660254037844387076, 1.000000000000000000, 0.8660254037844387076, 1.000000000000000000, 0.8660254037844387076, 1.000000000000000000, 0.8660254037844387076, 1.000000000000000000, 0.8660254037844387076, 1.000000000000000000, 0.8660254037844387076, 1.000000000000000000, 0.8660254037844387076, 1.000000000000000000, 0.8660254037844387076, 1.000000000000000000, 0.8660254037844387076, 1.000000000000000000, 0.8660254037844387076, 1.000000000000000000, 0.8660254037844387076, 1.000000000000000000, 0.8660254037844387076, 1.000000000000000000, 0.8660254037844387076, 1.000000000000000000, 0.8660254037844387076, 1.000000000000000000, 0.8660254037844387076, 1.000000000000000000, 0.8660254037844387076, 1.000000000000000000, 0.8660254037844387076, 1.000000000000000000, 0.8660254037844387076, 1.000000000000000000, 0.8660254037844387076, 1.000000000000000000, 0.8660254037844387076, 1.000000000000000000, 0.8660254037844387076, 1.000000000000000000, 0.8660254037844387076, 1.000000000000000000, 0.8660254037844387076, 1.000000000000000000, 0.8660254037844387076, 1.000000000000000000, 0.8660254037844387076, 1.000000000000000000, 0.8660254037844387076, 1.000000000000000000, 0.8660254037844387076, 1.000000000000000000, 0.8660254037844387076, 1.000000000000000000, 0.8660254037844387076, 1.000000000000000000, 0.8660254037844387076, 1.000000000000000000, 0.8660254037844387076, 1.000000000000000000, 0.8660254037844387076, 1.000000000000000000, 0.8660254037844387076, 1.000000000000000000, 0.8660254037844387076, 1.000000000000000000, 0.8660254037844387076, 1.000000000000000000, 0.8660254037844387076, 1.000000000000000000, 0.8660254037844387076, 1.000000000000000000, 0.8660254037844387076, 1.000000000000000000, 0.8660254037844387076, 1.000000000000000000, 0.8660254037844387076, 1.000000000000000000, 0.8660254037844387076, 1.000000000000000000, 0.8660254037844387076, 1.000000000000000000, 0.8660254037844387076, 1.000000000000000000, 0.8660254037844387076, 1.000000000000000000, 0.8660254037844387076, 1.000000000000000000, 0.8660254037844387076, 1.000000000000000000, 0.8660254037844387076, 1.000000000000000000, 0.8660254037844387076, 1.000000000000000000, 0.8660254037844387076, 1.000000000000000000, 0.8660254037844387076, 1.000000000000000000, 0.8660254037844387076, 1.000000000000000000, 0.8660254037844387076, 1.000000000000000000, 0.8660254037844387076, 1.000000000000000000, 0.8660254037844387076, 1.000000000000000000, 0.8660254037844387076, 1.000000000000000000, 0.8660254037844387076, 1.000000000000000000, 0.8660254037844387076, 1.000000000000000000, 0.8660254037844387076, 1.000000000000000000, 0.8660254037844387076, 1.000000000000000000, 0.8660254037844387076, 1.000000000000000000, 0.8660254037844387076, 1.000000000000000000, 0.8660254037844387076, 1.000000000000000000, 0.9211506902921580142, 0.9351132093492240394) ) ) 
 REPRESENTATION_ITEM ( '' )  SURFACE ( )  );
#2859=DIRECTION ( 'NONE',  ( -0.9928203230275512992, -0.1196152422706610319, -9.614813431917826478E-17 ) ) ;
#2860=DIRECTION ( 'NONE',  ( 0.9928203230275512992, 0.1196152422706610180, 4.006172263299093133E-17 ) ) ;
#2862=( BOUNDED_CURVE ( )  B_SPLINE_CURVE ( 2, ( #15273, #10994, #17940, #11083, #2774, #6670, #8294, #8030, #16647 ),
 .UNSPECIFIED., .F., .T. ) 
 B_SPLINE_CURVE_WITH_KNOTS ( ( 3, 2, 2, 2, 3 ),
 ( 0.5961538461538461453, 0.6025641025641025328, 0.6153846153846154188, 0.6282051282051281937, 0.6346153846153846922 ),
 .UNSPECIFIED. ) 
 CURVE ( )  GEOMETRIC_REPRESENTATION_ITEM ( )  RATIONAL_B_SPLINE_CURVE ( ( 0.9330127018922194093, 0.9330127018922194093, 1.000000000000000000, 0.8660254037844387076, 1.000000000000000000, 0.8660254037844387076, 1.000000000000000000, 0.9330127018922187432, 0.9330127018922192983 ) ) 
 REPRESENTATION_ITEM ( '' )  );
#2871=ORIENTED_EDGE ( 'NONE', *, *, #7022, .F. ) ;
#2879=CARTESIAN_POINT ( 'NONE',  ( 30.66050125466253107, -2.889050389913576655, -3.283357778048662023 ) ) ;
#2880=CARTESIAN_POINT ( 'NONE',  ( 32.29295089585318834, -5.599999616269981217, -3.283357778048667797 ) ) ;
#2883=CARTESIAN_POINT ( 'NONE',  ( 30.90769699326644826, -6.820963901304073929, -5.783357778048668685 ) ) ;
#2884=VECTOR ( 'NONE', #899, 1000.000000000000114 ) ;
#2885=CARTESIAN_POINT ( 'NONE',  ( 29.66420847303068697, -4.462897579762144851, -7.939653947423662039 ) ) ;
#2892=CYLINDRICAL_SURFACE ( 'NONE', #4161, 1.000000000000000000 ) ;
#2896=CARTESIAN_POINT ( 'NONE',  ( 29.99682221560115991, -1.914942061115552541, -5.783357778048658027 ) ) ;
#2898=DIRECTION ( 'NONE',  ( 0.6951637808321680101, -0.2969442527608454063, 0.6546536707079773088 ) ) ;
#2899=CARTESIAN_POINT ( 'NONE',  ( 27.36943512155133362, -2.558652073080304845, -4.533357778048659803 ) ) ;
#2909=CARTESIAN_POINT ( 'NONE',  ( 30.15026255541241440, -6.285249260098253465, -4.705209693361168455 ) ) ;
#2913=DIRECTION ( 'NONE',  ( -0.1196152422706610735, 0.9928203230275511881, 0.000000000000000000 ) ) ;
#2918=ORIENTED_EDGE ( 'NONE', *, *, #11232, .T. ) ;
#2925=LINE ( 'NONE', #209, #286 ) ;
#2927=CIRCLE ( 'NONE', #8724, 0.9999999999999995559 ) ;
#2929=CARTESIAN_POINT ( 'NONE',  ( 33.32864623319426300, -4.021405196597508613, -3.283357778048664688 ) ) ;
#2942=( NAMED_UNIT ( * ) PLANE_ANGLE_UNIT ( ) SI_UNIT ( $, .RADIAN. ) );
#2947=VECTOR ( 'NONE', #5945, 1000.000000000000114 ) ;
#2954=CARTESIAN_POINT ( 'NONE',  ( 31.66930131758986988, -2.967382423816733894, -3.627061608673662008 ) ) ;
#2961=CIRCLE ( 'NONE', #15416, 3.000000000000001332 ) ;
#2964=ORIENTED_EDGE ( 'NONE', *, *, #16092, .F. ) ;
#2974=DIRECTION ( 'NONE',  ( -0.1196152422706610735, 0.9928203230275511881, 0.000000000000000000 ) ) ;
#2976=CARTESIAN_POINT ( 'NONE',  ( 26.49878054387835746, -2.963357534503999968, -4.705209693361160461 ) ) ;
#2979=CARTESIAN_POINT ( 'NONE',  ( 29.39961944441754227, -3.040961747597316300, -3.283357778048662023 ) ) ;
#2982=CARTESIAN_POINT ( 'NONE',  ( 46.62628598016694070, -0.4028612494373206565, -5.783357778048661579 ) ) ;
#2984=CARTESIAN_POINT ( 'NONE',  ( 32.54050588463559990, -2.235448945602741766, -6.861505862736159145 ) ) ;
#2990=VERTEX_POINT ( 'NONE', #17070 ) ;
#2997=CARTESIAN_POINT ( 'NONE',  ( 32.52441275490655670, -6.636378442139655220, -5.783357778048663356 ) ) ;
#2998=CARTESIAN_POINT ( 'NONE',  ( 32.96459815279162342, -1.884545423566157174, -4.533357778048659803 ) ) ;
#2999=CARTESIAN_POINT ( 'NONE',  ( 30.23341599105502908, -5.648260380436597394, -7.939653947423664704 ) ) ;
#3013=CARTESIAN_POINT ( 'NONE',  ( 28.86293393808771057, -2.678523738846987357, -4.705209693361161349 ) ) ;
#3016=DIRECTION ( 'NONE',  ( 0.9928203230275512992, 0.1196152422706610180, 4.006172263299093133E-17 ) ) ;
#3026=CARTESIAN_POINT ( 'NONE',  ( 31.66250999073069750, -5.675955295111851484, -3.283357778048667797 ) ) ;
#3027=ADVANCED_FACE ( 'NONE', ( #3958 ), #13572, .T. ) ;
#3036=SURFACE_STYLE_FILL_AREA ( #7033 ) ;
#3041=CARTESIAN_POINT ( 'NONE',  ( 29.74794773085836397, -1.934729659147405689, -5.113484796970855228 ) ) ;
#3042=EDGE_CURVE ( 'NONE', #4105, #16322, #12301, .T. ) ;
#3048=CARTESIAN_POINT ( 'NONE',  ( 32.95662993491455950, -6.574107945067995118, -5.783357778048669573 ) ) ;
#3061=CYLINDRICAL_SURFACE ( 'NONE', #4869, 2.500000000000001776 ) ;
#3065=CARTESIAN_POINT ( 'NONE',  ( 33.59503905791412137, -1.808589744724287129, -4.533357778048659803 ) ) ;
#3066=CARTESIAN_POINT ( 'NONE',  ( 32.77257290155422709, -2.834459985843461816, -3.627061608673662896 ) ) ;
#3070=CARTESIAN_POINT ( 'NONE',  ( 31.39792096211754924, -4.254019462947003838, -7.939653947423662039 ) ) ;
#3073=CARTESIAN_POINT ( 'NONE',  ( 26.63030083514515312, -6.709335133632020387, -6.861505862736167138 ) ) ;
#3084=CARTESIAN_POINT ( 'NONE',  ( 33.76207435632690590, -3.969185667289998332, -3.627061608673664672 ) ) ;
#3087=ORIENTED_EDGE ( 'NONE', *, *, #12395, .F. ) ;
#3089=CARTESIAN_POINT ( 'NONE',  ( 27.95866967485789090, -6.122194908100387245, -3.283357778048667797 ) ) ;
#3108=DIRECTION ( 'NONE',  ( 0.9928203230275510771, 0.1196152422706609902, 4.006172263299092517E-17 ) ) ;
#3111=CARTESIAN_POINT ( 'NONE',  ( 32.19529564017040002, -1.250324391365404741, -5.783357778048658027 ) ) ;
#3120=DIRECTION ( 'NONE',  ( 0.1196152422706587976, -0.9928203230275515212, 1.866876274697368064E-15 ) ) ;
#3125=CARTESIAN_POINT ( 'NONE',  ( 30.54048978798443059, -6.538043363838207611, -4.533357778048668685 ) ) ;
#3131=CARTESIAN_POINT ( 'NONE',  ( 32.19919549706052209, -6.038393303862174655, -4.705209693361169343 ) ) ;
#3146=CIRCLE ( 'NONE', #3729, 2.001963570546864801 ) ;
#3150=CARTESIAN_POINT ( 'NONE',  ( 25.61697401368257587, -3.496695820648536568, -3.283357778048662023 ) ) ;
#3151=CARTESIAN_POINT ( 'NONE',  ( 33.40745134805642635, -4.011910736534825439, -3.283357778048664688 ) ) ;
#3154=CARTESIAN_POINT ( 'NONE',  ( 30.75425665345519732, -2.450656702321377001, -4.705209693361161349 ) ) ;
#3155=CARTESIAN_POINT ( 'NONE',  ( 26.39823381822652593, -6.110324093391315436, -3.627061608673668225 ) ) ;
#3158=ORIENTED_EDGE ( 'NONE', *, *, #9234, .T. ) ;
#3166=CARTESIAN_POINT ( 'NONE',  ( 31.66930131758986988, -2.967382423816733894, -3.627061608673662008 ) ) ;
#3170=VECTOR ( 'NONE', #16599, 1000.000000000000227 ) ;
#3182=VECTOR ( 'NONE', #1774, 1000.000000000000114 ) ;
#3187=ORIENTED_EDGE ( 'NONE', *, *, #3576, .T. ) ;
#3194=CARTESIAN_POINT ( 'NONE',  ( 26.58890374069123652, -3.379597482641427231, -8.283357778048660691 ) ) ;
#3199=CARTESIAN_POINT ( 'NONE',  ( 32.43181250335191379, -6.310176327312596811, -4.533357778048668685 ) ) ;
#3200=CARTESIAN_POINT ( 'NONE',  ( 29.07687923786957285, -2.352938776424351008, -7.033357778048658027 ) ) ;
#3209=ADVANCED_FACE ( 'NONE', ( #8299 ), #16934, .T. ) ;
#3216=CARTESIAN_POINT ( 'NONE',  ( 29.95125523467787332, -2.974500528818129652, -3.283357778048662023 ) ) ;
#3219=CARTESIAN_POINT ( 'NONE',  ( 41.90164972253718645, -2.988527579590353422, -5.783357778048662468 ) ) ;
#3221=FACE_BOUND ( 'NONE', #16571, .T. ) ;
#3222=CARTESIAN_POINT ( 'NONE',  ( 33.23365877489121090, -6.550928303235100891, -5.783357778048663356 ) ) ;
#3224=CARTESIAN_POINT ( 'NONE',  ( 26.85044460880409645, -7.319979551716484067, -5.783357778048668685 ) ) ;
#3244=CARTESIAN_POINT ( 'NONE',  ( 25.33925079868512498, -2.076342398563292058, -5.783357778048658027 ) ) ;
#3249=CARTESIAN_POINT ( 'NONE',  ( 30.01874226414561875, -2.539271660970221944, -6.861505862736159145 ) ) ;
#3255=ORIENTED_EDGE ( 'NONE', *, *, #12421, .T. ) ;
#3265=CARTESIAN_POINT ( 'NONE',  ( 32.93470988637010066, -5.949778345213319497, -6.861505862736167138 ) ) ;
#3267=DIRECTION ( 'NONE',  ( 0.1196152422706597829, -0.9928203230275514102, 0.000000000000000000 ) ) ;
#3284=ORIENTED_EDGE ( 'NONE', *, *, #10028, .F. ) ;
#3286=ORIENTED_EDGE ( 'NONE', *, *, #1913, .F. ) ;
#3297=ORIENTED_EDGE ( 'NONE', *, *, #7038, .F. ) ;
#3298=CARTESIAN_POINT ( 'NONE',  ( 29.95125523467787687, -2.974500528818130096, -3.283357778048662023 ) ) ;
#3299=CARTESIAN_POINT ( 'NONE',  ( 39.19942832275109623, -5.640193629429878897, -9.783357778048662468 ) ) ;
#3303=CARTESIAN_POINT ( 'NONE',  ( 30.74004950963507810, -6.851358974801540214, -6.453230759126470595 ) ) ;
#3305=ORIENTED_EDGE ( 'NONE', *, *, #8060, .T. ) ;
#3313=DIRECTION ( 'NONE',  ( 0.9928203230275512992, 0.1196152422706610180, 4.006172263299093133E-17 ) ) ;
#3318=CARTESIAN_POINT ( 'NONE',  ( 32.04575515724926760, -1.668086104879473730, -5.783357778048658027 ) ) ;
#3325=CARTESIAN_POINT ( 'NONE',  ( 25.93714794488954212, -2.393855775999666591, -5.783357778048658027 ) ) ;
#3329=CARTESIAN_POINT ( 'NONE',  ( 42.32364987186199556, -2.937684895442014277, -5.783357778048662468 ) ) ;
#3330=ORIENTED_EDGE ( 'NONE', *, *, #6121, .T. ) ;
#3335=CARTESIAN_POINT ( 'NONE',  ( 26.27749392786457250, -6.324743385012029151, -8.283357778048662468 ) ) ;
#3338=CARTESIAN_POINT ( 'NONE',  ( 28.88938074516742205, -6.437160617781993999, -4.705209693361168455 ) ) ;
#3340=CARTESIAN_POINT ( 'NONE',  ( 27.23882169172318513, -6.009049854935478052, -7.939653947423662927 ) ) ;
#3342=VERTEX_POINT ( 'NONE', #6301 ) ;
#3348=CARTESIAN_POINT ( 'NONE',  ( 46.62628598016694781, -0.4028612494373219333, -5.783357778048661579 ) ) ;
#3351=CARTESIAN_POINT ( 'NONE',  ( 33.44685390376565692, -4.007163506710925027, -7.939653947423662039 ) ) ;
#3352=CARTESIAN_POINT ( 'NONE',  ( 30.61177514885986639, -5.802548093181622235, -8.283357778048664244 ) ) ;
#3360=VERTEX_POINT ( 'NONE', #6213 ) ;
#3372=DIRECTION ( 'NONE',  ( -0.1196152422706609625, 0.9928203230275510771, 0.000000000000000000 ) ) ;
#3381=CARTESIAN_POINT ( 'NONE',  ( 29.35089333861488115, -5.954459450865362768, -8.283357778048662468 ) ) ;
#3387=CARTESIAN_POINT ( 'NONE',  ( 26.01652455409633902, -4.902371455920926380, -5.783357778048663356 ) ) ;
#3400=CARTESIAN_POINT ( 'NONE',  ( 29.80442540930208750, -6.953886339277345563, -5.783357778048669573 ) ) ;
#3406=CARTESIAN_POINT ( 'NONE',  ( 25.62757597683262034, -3.695291012717980994, -7.939653947423660263 ) ) ;
#3419=CARTESIAN_POINT ( 'NONE',  ( 27.32822876973539294, -6.198150586942257512, -3.283357778048667797 ) ) ;
#3423=CARTESIAN_POINT ( 'NONE',  ( 26.88845778707760914, -3.543379655034240905, -7.939653947423660263 ) ) ;
#3439=CARTESIAN_POINT ( 'NONE',  ( 32.95662993491455950, -6.574107945067995118, -5.783357778048669573 ) ) ;
#3444=CARTESIAN_POINT ( 'NONE',  ( 27.32822876973539294, -6.198150586942257512, -3.283357778048667797 ) ) ;
#3445=( BOUNDED_CURVE ( )  B_SPLINE_CURVE ( 2, ( #484, #10168, #10070, #5993, #11519, #6090, #17088, #1857, #15720 ),
 .UNSPECIFIED., .F., .T. ) 
 B_SPLINE_CURVE_WITH_KNOTS ( ( 3, 2, 2, 2, 3 ),
 ( 0.5961538461538461453, 0.6025641025641025328, 0.6153846153846154188, 0.6282051282051281937, 0.6346153846153846922 ),
 .UNSPECIFIED. ) 
 CURVE ( )  GEOMETRIC_REPRESENTATION_ITEM ( )  RATIONAL_B_SPLINE_CURVE ( ( 0.9330127018922194093, 0.9330127018922194093, 1.000000000000000000, 0.8660254037844387076, 1.000000000000000000, 0.8660254037844387076, 1.000000000000000000, 0.9330127018922187432, 0.9330127018922192983 ) ) 
 REPRESENTATION_ITEM ( '' )  );
#3451=CARTESIAN_POINT ( 'NONE',  ( 32.29974222271236073, -2.891426744974864071, -3.627061608673662008 ) ) ;
#3462=CARTESIAN_POINT ( 'NONE',  ( 29.18195272205665347, -2.340279496617377664, -4.533357778048659803 ) ) ;
#3463=CARTESIAN_POINT ( 'NONE',  ( 32.87199790123699472, -1.558343308739095656, -5.783357778048663356 ) ) ;
#3472=CARTESIAN_POINT ( 'NONE',  ( 27.92107091181166467, -2.492190854301117753, -4.533357778048659803 ) ) ;
#3478=CARTESIAN_POINT ( 'NONE',  ( 26.95740407890011170, -7.307093047852763590, -6.453230759126468818 ) ) ;
#3481=LINE ( 'NONE', #15633, #9615 ) ;
#3492=DIRECTION ( 'NONE',  ( 0.9928203230275512992, 0.1196152422706610180, 4.006172263299093133E-17 ) ) ;
#3493=CARTESIAN_POINT ( 'NONE',  ( 30.28142597461332741, -2.507623461452779701, -4.705209693361160461 ) ) ;
#3499=CARTESIAN_POINT ( 'NONE',  ( 26.87106449706838873, -6.053357334259913181, -3.627061608673667781 ) ) ;
#3503=CARTESIAN_POINT ( 'NONE',  ( 27.45957062324739084, -6.182326487390971792, -8.283357778048664244 ) ) ;
#3511=CARTESIAN_POINT ( 'NONE',  ( 32.75517961154501023, -5.344437665069116328, -7.939653947423664704 ) ) ;
#3514=CARTESIAN_POINT ( 'NONE',  ( 26.45077056032005913, -6.103994453487816330, -7.939653947423664704 ) ) ;
#3519=EDGE_CURVE ( 'NONE', #16712, #3946, #9186, .T. ) ;
#3520=VERTEX_POINT ( 'NONE', #14744 ) ;
#3526=( BOUNDED_CURVE ( )  B_SPLINE_CURVE ( 2, ( #5489, #4157, #17875, #5399, #17619, #9654, #9485, #15025, #2445 ),
 .UNSPECIFIED., .F., .T. ) 
 B_SPLINE_CURVE_WITH_KNOTS ( ( 3, 2, 2, 2, 3 ),
 ( 0.3269230769230769273, 0.3333333333333333148, 0.3461538461538461453, 0.3589743589743589758, 0.3653846153846154188 ),
 .UNSPECIFIED. ) 
 CURVE ( )  GEOMETRIC_REPRESENTATION_ITEM ( )  RATIONAL_B_SPLINE_CURVE ( ( 0.9330127018922194093, 0.9330127018922194093, 1.000000000000000000, 0.8660254037844387076, 1.000000000000000000, 0.8660254037844387076, 1.000000000000000000, 0.9330127018922190762, 0.9330127018922194093 ) ) 
 REPRESENTATION_ITEM ( '' )  );
#3528=CARTESIAN_POINT ( 'NONE',  ( 29.81991338116587542, -2.990324628369393611, -8.283357778048660691 ) ) ;
#3530=CARTESIAN_POINT ( 'NONE',  ( 29.03376756790819613, -4.538853258604016006, -7.939653947423662039 ) ) ;
#3532=CARTESIAN_POINT ( 'NONE',  ( 38.15053902264412500, -1.114360604510109765, -9.783357778048662468 ) ) ;
#3536=CARTESIAN_POINT ( 'NONE',  ( 31.05948030073166066, -1.776715885202022394, -5.783357778048662468 ) ) ;
#3539=ORIENTED_EDGE ( 'NONE', *, *, #3647, .T. ) ;
#3544=CARTESIAN_POINT ( 'NONE',  ( 31.69574812466957781, -6.726019302751734763, -5.783357778048669573 ) ) ;
#3553=AXIS2_PLACEMENT_3D ( 'NONE', #4576, #12737, #4311 ) ;
#3555=( BOUNDED_CURVE ( )  B_SPLINE_CURVE ( 2, ( #7000, #10467, #2479, #6636, #6820, #8186, #2562, #21, #15163 ),
 .UNSPECIFIED., .F., .T. ) 
 B_SPLINE_CURVE_WITH_KNOTS ( ( 3, 2, 2, 2, 3 ),
 ( 0.09615384615384617306, 0.1025641025641025605, 0.1153846153846153910, 0.1282051282051281937, 0.1346153846153846367 ),
 .UNSPECIFIED. ) 
 CURVE ( )  GEOMETRIC_REPRESENTATION_ITEM ( )  RATIONAL_B_SPLINE_CURVE ( ( 0.9330127018922194093, 0.9330127018922196314, 1.000000000000000000, 0.8660254037844387076, 1.000000000000000000, 0.8660254037844387076, 1.000000000000000000, 0.9330127018922190762, 0.9330127018922194093 ) ) 
 REPRESENTATION_ITEM ( '' )  );
#3557=ORIENTED_EDGE ( 'NONE', *, *, #15558, .T. ) ;
#3567=CARTESIAN_POINT ( 'NONE',  ( 25.95642634701329499, -4.403549397486667516, -3.686412874245489135 ) ) ;
#3568=CARTESIAN_POINT ( 'NONE',  ( 37.96876116389215383, 4.574485896386907058, -9.283357778048655362 ) ) ;
#3572=CARTESIAN_POINT ( 'NONE',  ( 26.70901672940806648, -4.818939824437135755, -8.283357778048662468 ) ) ;
#3573=CARTESIAN_POINT ( 'NONE',  ( 33.38562051666750818, -5.268481986227246949, -7.939653947423662927 ) ) ;
#3575=AXIS2_PLACEMENT_3D ( 'NONE', #5095, #17575, #9272 ) ;
#3576=EDGE_CURVE ( 'NONE', #10379, #15769, #6867, .T. ) ;
#3582=ORIENTED_EDGE ( 'NONE', *, *, #16826, .F. ) ;
#3584=FACE_OUTER_BOUND ( 'NONE', #16093, .T. ) ;
#3586=DIRECTION ( 'NONE',  ( 0.1196152422706596996, -0.9928203230275514102, 0.000000000000000000 ) ) ;
#3593=CARTESIAN_POINT ( 'NONE',  ( 28.39010325924584421, -2.735490497978389612, -4.705209693361160461 ) ) ;
#3611=CARTESIAN_POINT ( 'NONE',  ( 32.04158527077989760, -6.057382223572642665, -4.705209693361168455 ) ) ;
#3613=CARTESIAN_POINT ( 'NONE',  ( 31.66176685062031027, -1.704152250161192539, -6.453230759126468818 ) ) ;
#3614=CARTESIAN_POINT ( 'NONE',  ( 27.51889869220010354, -3.467423976192371082, -7.939653947423660263 ) ) ;
#3623=CARTESIAN_POINT ( 'NONE',  ( 25.71748644841968456, -2.420320648352046078, -5.783357778048663356 ) ) ;
#3627=EDGE_CURVE ( 'NONE', #17548, #397, #2269, .T. ) ;
#3630=CARTESIAN_POINT ( 'NONE',  ( 28.71854711534694715, -4.576831098024959132, -3.627061608673664672 ) ) ;
#3639=CARTESIAN_POINT ( 'NONE',  ( 32.82963640218302004, -5.962437625020304388, -4.705209693361169343 ) ) ;
#3647=EDGE_CURVE ( 'NONE', #10267, #11388, #12897, .T. ) ;
#3649=LINE ( 'NONE', #8905, #10490 ) ;
#3657=CARTESIAN_POINT ( 'NONE',  ( 27.78220930431293922, -1.782014143258494832, -5.783357778048658027 ) ) ;
#3658=CARTESIAN_POINT ( 'NONE',  ( 32.54503264317084188, -5.369756224683081669, -3.627061608673667781 ) ) ;
#3660=CARTESIAN_POINT ( 'NONE',  ( 30.25524682244395436, -4.391689130744175884, -3.283357778048664688 ) ) ;
#3663=DIRECTION ( 'NONE',  ( -0.1196152422706609625, 0.9928203230275510771, -4.694733121053619507E-17 ) ) ;
#3670=CARTESIAN_POINT ( 'NONE',  ( 26.56758885001203652, -2.317900097157796324, -5.783357778048670461 ) ) ;
#3671=CARTESIAN_POINT ( 'NONE',  ( 28.91547068018125799, -2.672194098943493135, -6.861505862736158257 ) ) ;
#3689=CARTESIAN_POINT ( 'NONE',  ( 32.54503264317084188, -5.369756224683081669, -3.627061608673667781 ) ) ;
#3692=CARTESIAN_POINT ( 'NONE',  ( 28.34209327568754233, -5.876127416962207306, -7.939653947423664704 ) ) ;
#3693=EDGE_CURVE ( 'NONE', #9123, #3859, #2034, .T. ) ;
#3707=CARTESIAN_POINT ( 'NONE',  ( 30.18087924896149588, -5.654590020340094725, -3.627061608673668225 ) ) ;
#3708=DIRECTION ( 'NONE',  ( 0.05980762113533059227, -0.4964101615137756496, -0.8660254037844385966 ) ) ;
#3709=CARTESIAN_POINT ( 'NONE',  ( 31.74131510559286085, -5.666460835049168310, -3.283357778048667797 ) ) ;
#3717=CARTESIAN_POINT ( 'NONE',  ( 31.43723430067123914, -2.368371383576012956, -6.861505862736158257 ) ) ;
#3729=AXIS2_PLACEMENT_3D ( 'NONE', #6931, #12464, #12199 ) ;
#3738=CARTESIAN_POINT ( 'NONE',  ( 28.55151181693415907, -2.416235175459247486, -4.533357778048659803 ) ) ;
#3740=CARTESIAN_POINT ( 'NONE',  ( 30.64918316926811315, -2.463315982128351678, -6.861505862736159145 ) ) ;
#3744=ADVANCED_FACE ( 'NONE', ( #9004 ), #1947, .T. ) ;
#3746=DIRECTION ( 'NONE',  ( 0.05980762113533044655, -0.4964101615137759826, 0.8660254037844383745 ) ) ;
#3756=ORIENTED_EDGE ( 'NONE', *, *, #10540, .F. ) ;
#3762=CARTESIAN_POINT ( 'NONE',  ( 31.45915434921569798, -2.992700983430681028, -7.939653947423660263 ) ) ;
#3764=CARTESIAN_POINT ( 'NONE',  ( 33.42946061375642586, -6.517141185936593750, -5.783357778048668685 ) ) ;
#3774=CARTESIAN_POINT ( 'NONE',  ( 33.18300801526289234, -6.557030719496743210, -6.453230759126470595 ) ) ;
#3777=DIRECTION ( 'NONE',  ( -0.05980762113533043267, 0.4964101615137759826, -0.8660254037844384856 ) ) ;
#3805=CARTESIAN_POINT ( 'NONE',  ( 29.14753769709988518, -3.271205139184214516, -3.627061608673662008 ) ) ;
#3806=CARTESIAN_POINT ( 'NONE',  ( 38.69874410340102600, -1.484456793942448449, -2.033357778048666464 ) ) ;
#3808=CARTESIAN_POINT ( 'NONE',  ( 32.55182397003001427, -2.661183353387966299, -3.283357778048662023 ) ) ;
#3810=CARTESIAN_POINT ( 'NONE',  ( 26.85044460880409645, -7.319979551716484067, -5.783357778048668685 ) ) ;
#3818=CARTESIAN_POINT ( 'NONE',  ( 46.86575133767496482, -2.390451368237048513, -5.783357778048662468 ) ) ;
#3823=EDGE_CURVE ( 'NONE', #2767, #7401, #507, .T. ) ;
#3824=DIRECTION ( 'NONE',  ( -0.1196152422706598106, 0.9928203230275514102, 0.000000000000000000 ) ) ;
#3826=CARTESIAN_POINT ( 'NONE',  ( 28.75424055680402802, -6.753251120556833520, -7.033357778048666908 ) ) ;
#3839=CARTESIAN_POINT ( 'NONE',  ( 32.77257290155422709, -2.834459985843462260, -3.627061608673662896 ) ) ;
#3844=ADVANCED_FACE ( 'NONE', ( #8621 ), #16981, .T. ) ;
#3855=CARTESIAN_POINT ( 'NONE',  ( 28.54354359905709870, -7.105797696961086096, -5.783357778048669573 ) ) ;
#3859=VERTEX_POINT ( 'NONE', #14345 ) ;
#3865=DIRECTION ( 'NONE',  ( 0.9928203230275512992, 0.1196152422706610180, 4.006172263299093133E-17 ) ) ;
#3872=LINE ( 'NONE', #3952, #6363 ) ;
#3884=DIRECTION ( 'NONE',  ( -0.1196152422706610735, 0.9928203230275511881, 0.000000000000000000 ) ) ;
#3889=CARTESIAN_POINT ( 'NONE',  ( 30.19827253897071273, -3.144612341114420673, -7.939653947423660263 ) ) ;
#3890=CARTESIAN_POINT ( 'NONE',  ( 26.18940075748478691, -6.337263906362392341, -7.823530922983556124 ) ) ;
#3895=SURFACE_STYLE_FILL_AREA ( #12319 ) ;
#3897=CARTESIAN_POINT ( 'NONE',  ( 30.30787278169304244, -6.266260340387784566, -4.705209693361169343 ) ) ;
#3912=CARTESIAN_POINT ( 'NONE',  ( 28.48022645605872327, -3.151730446115816875, -8.283357778048660691 ) ) ;
#3918=CARTESIAN_POINT ( 'NONE',  ( 26.17715024865825768, -6.235583268514400146, -3.900143082538624739 ) ) ;
#3923=CARTESIAN_POINT ( 'NONE',  ( 32.64557936882268052, -2.222789665795767089, -4.705209693361161349 ) ) ;
#3930=ORIENTED_EDGE ( 'NONE', *, *, #7071, .T. ) ;
#3936=DIRECTION ( 'NONE',  ( 0.9928203230275512992, 0.1196152422706610180, 4.006172263299093133E-17 ) ) ;
#3937=CARTESIAN_POINT ( 'NONE',  ( 27.65911562847151117, -5.958412735707574015, -3.627061608673668225 ) ) ;
#3945=ADVANCED_FACE ( 'NONE', ( #12178 ), #16019, .T. ) ;
#3946=VERTEX_POINT ( 'NONE', #2412 ) ;
#3952=CARTESIAN_POINT ( 'NONE',  ( 39.19942832275109623, -5.640193629429882449, -1.783357778048662690 ) ) ;
#3958=FACE_OUTER_BOUND ( 'NONE', #13769, .T. ) ;
#3967=CARTESIAN_POINT ( 'NONE',  ( 38.74759774169763915, -1.889947633019406270, 3.759232513472238413 ) ) ;
#3974=CARTESIAN_POINT ( 'NONE',  ( 25.76326615456878244, -3.051972493152843580, -6.861505862736158257 ) ) ;
#3976=CARTESIAN_POINT ( 'NONE',  ( 26.31556265977298992, -7.384422263489805793, -5.783357778048663356 ) ) ;
#3978=VECTOR ( 'NONE', #14739, 1000.000000000000227 ) ;
#3980=( LENGTH_UNIT ( ) NAMED_UNIT ( * ) SI_UNIT ( .MILLI., .METRE. ) );
#3982=CARTESIAN_POINT ( 'NONE',  ( 27.75966235412334981, -2.811446176820259879, -4.705209693361160461 ) ) ;
#3987=VERTEX_POINT ( 'NONE', #3670 ) ;
#3991=CARTESIAN_POINT ( 'NONE',  ( 26.31556265977298992, -7.384422263489805793, -5.783357778048663356 ) ) ;
#3992=CARTESIAN_POINT ( 'NONE',  ( 28.35948656569675919, -3.366149737736551906, -3.627061608673662896 ) ) ;
#3993=CARTESIAN_POINT ( 'NONE',  ( 28.72045243349238675, -6.030415129707233035, -8.283357778048664244 ) ) ;
#3999=VECTOR ( 'NONE', #7881, 1000.000000000000114 ) ;
#4006=DIRECTION ( 'NONE',  ( -0.05980762113533058533, 0.4964101615137755386, 0.8660254037844385966 ) ) ;
#4007=CARTESIAN_POINT ( 'NONE',  ( 29.60297508593253468, -5.724216059278466773, -7.939653947423662927 ) ) ;
#4015=EDGE_CURVE ( 'NONE', #17192, #17584, #4928, .T. ) ;
#4022=CARTESIAN_POINT ( 'NONE',  ( 33.83155592109562804, -6.868441680671474536, -5.783357778048669573 ) ) ;
#4028=CARTESIAN_POINT ( 'NONE',  ( 36.48725301720441649, 2.437776833296281698, -5.783357778048662468 ) ) ;
#4032=FACE_OUTER_BOUND ( 'NONE', #11264, .T. ) ;
#4036=DIRECTION ( 'NONE',  ( 0.9928203230275510771, 0.1196152422706609902, 4.006172263299092517E-17 ) ) ;
#4043=DIRECTION ( 'NONE',  ( 0.9928203230275512992, 0.1196152422706610180, 4.006172263299093133E-17 ) ) ;
#4052=CARTESIAN_POINT ( 'NONE',  ( 29.45101334415624095, -7.006662376286320715, -5.783357778048657138 ) ) ;
#4059=CARTESIAN_POINT ( 'NONE',  ( 27.25621498173240198, -3.499072175709823984, -3.627061608673662008 ) ) ;
#4062=CARTESIAN_POINT ( 'NONE',  ( 31.20090818012769773, -4.277755612481361602, -8.283357778048662468 ) ) ;
#4068=CIRCLE ( 'NONE', #6967, 2.499999999999999556 ) ;
#4070=CARTESIAN_POINT ( 'NONE',  ( 27.65458886993626564, -2.824105456627233224, -6.861505862736158257 ) ) ;
#4074=EDGE_LOOP ( 'NONE', ( #7114, #11534, #12477, #8643 ) ) ;
#4077=LINE ( 'NONE', #15144, #3170 ) ;
#4079=CARTESIAN_POINT ( 'NONE',  ( 27.60205212784272177, -2.830435096530727446, -4.705209693361161349 ) ) ;
#4084=DIRECTION ( 'NONE',  ( 0.9928203230275510771, 0.1196152422706609902, 4.006172263299092517E-17 ) ) ;
#4088=ORIENTED_EDGE ( 'NONE', *, *, #11765, .F. ) ;
#4091=EDGE_CURVE ( 'NONE', #13220, #14372, #2574, .T. ) ;
#4093=CARTESIAN_POINT ( 'NONE',  ( 25.71748644841968456, -2.420320648352046078, -5.783357778048663356 ) ) ;
#4096=CARTESIAN_POINT ( 'NONE',  ( 29.49337484321020497, -2.602568060005117090, -4.705209693361161349 ) ) ;
#4105=VERTEX_POINT ( 'NONE', #9623 ) ;
#4115=CARTESIAN_POINT ( 'NONE',  ( 26.65222088368961195, -7.333664733486695120, -5.783357778048669573 ) ) ;
#4125=AXIS2_PLACEMENT_3D ( 'NONE', #15186, #16548, #8289 ) ;
#4128=CARTESIAN_POINT ( 'NONE',  ( 27.22618411036838637, -2.238552374514887866, -5.113484796970851676 ) ) ;
#4145=AXIS2_PLACEMENT_3D ( 'NONE', #11905, #7929, #17488 ) ;
#4146=VECTOR ( 'NONE', #12919, 1000.000000000000114 ) ;
#4153=FACE_OUTER_BOUND ( 'NONE', #921, .T. ) ;
#4157=CARTESIAN_POINT ( 'NONE',  ( 30.95252083063564896, -1.789602389065743981, -6.453230759126464378 ) ) ;
#4158=LINE ( 'NONE', #13586, #15914 ) ;
#4160=CARTESIAN_POINT ( 'NONE',  ( 26.03726795043090547, -3.446058701420613879, -8.283357778048660691 ) ) ;
#4161=AXIS2_PLACEMENT_3D ( 'NONE', #16875, #8328, #269 ) ;
#4163=CARTESIAN_POINT ( 'NONE',  ( 29.15568435273173264, -2.343444316361667834, -7.033357778048658027 ) ) ;
#4169=CARTESIAN_POINT ( 'NONE',  ( 28.89355063163679915, -2.047864499088824175, -5.783357778048658915 ) ) ;
#4171=CARTESIAN_POINT ( 'NONE',  ( 41.90164972253718645, -2.988527579590353422, -5.783357778048662468 ) ) ;
#4179=CARTESIAN_POINT ( 'NONE',  ( 28.76917853929504432, -3.116917426439186123, -3.283357778048662023 ) ) ;
#4180=CARTESIAN_POINT ( 'NONE',  ( 27.61527553138257574, -4.709753535998224550, -7.939653947423662039 ) ) ;
#4181=CARTESIAN_POINT ( 'NONE',  ( 26.24741491880506672, -3.420740141806666301, -3.283357778048662023 ) ) ;
#4190=CARTESIAN_POINT ( 'NONE',  ( 27.62849893492243325, -6.589071975465733644, -4.705209693361168455 ) ) ;
#4196=ORIENTED_EDGE ( 'NONE', *, *, #2189, .F. ) ;
#4199=EDGE_CURVE ( 'NONE', #4757, #4277, #8638, .T. ) ;
#4206=CARTESIAN_POINT ( 'NONE',  ( 27.63266882139180680, -2.199775856772564708, -5.783357778048658027 ) ) ;
#4207=CARTESIAN_POINT ( 'NONE',  ( 41.90164972253716513, -2.988527579590351646, -5.783357778048662468 ) ) ;
#4208=ORIENTED_EDGE ( 'NONE', *, *, #4934, .T. ) ;
#4211=CARTESIAN_POINT ( 'NONE',  ( 37.87429945334753256, 1.178459718517443022, -5.783357778048661579 ) ) ;
#4216=DIRECTION ( 'NONE',  ( 0.5595328448060640225, 0.8288081777970298658, -3.349091179051939016E-15 ) ) ;
#4217=ORIENTED_EDGE ( 'NONE', *, *, #5069, .F. ) ;
#4241=CARTESIAN_POINT ( 'NONE',  ( 26.41562710823574278, -3.600346414165641828, -7.939653947423660263 ) ) ;
#4243=APPLICATION_CONTEXT ( 'automotive_design' ) ;
#4244=CARTESIAN_POINT ( 'NONE',  ( 29.42969845347704450, -5.944964990802679594, -8.283357778048662468 ) ) ;
#4245=CARTESIAN_POINT ( 'NONE',  ( 31.84257795004536007, -2.746633492292519296, -3.283357778048662023 ) ) ;
#4249=CARTESIAN_POINT ( 'NONE',  ( 31.51169109130924184, -2.986371343527201905, -3.627061608673662896 ) ) ;
#4251=CARTESIAN_POINT ( 'NONE',  ( 27.86926259684567597, -5.933094176093607786, -7.939653947423662927 ) ) ;
#4260=AXIS2_PLACEMENT_3D ( 'NONE', #14151, #8721, #12887 ) ;
#4263=CARTESIAN_POINT ( 'NONE',  ( 28.10549950023366961, -2.142809097641162897, -5.783357778048658027 ) ) ;
#4265=DIRECTION ( 'NONE',  ( 0.9928203230275512992, 0.1196152422706610180, 4.006172263299093133E-17 ) ) ;
#4267=EDGE_CURVE ( 'NONE', #14747, #7654, #8909, .T. ) ;
#4275=CARTESIAN_POINT ( 'NONE',  ( 27.73357241910951743, -6.576412695658750529, -6.861505862736166250 ) ) ;
#4277=VERTEX_POINT ( 'NONE', #7200 ) ;
#4279=CARTESIAN_POINT ( 'NONE',  ( 28.19013153391124860, -7.158573733970061248, -5.783357778048657138 ) ) ;
#4289=CARTESIAN_POINT ( 'NONE',  ( 29.81239362717914787, -2.264323817775507397, -4.533357778048659803 ) ) ;
#4291=ORIENTED_EDGE ( 'NONE', *, *, #785, .F. ) ;
#4311=DIRECTION ( 'NONE',  ( 0.1196152422706608098, -0.9928203230275511881, 0.000000000000000000 ) ) ;
#4327=CARTESIAN_POINT ( 'NONE',  ( 27.15566825608056689, -6.646038734597135011, -4.705209693361169343 ) ) ;
#4329=CARTESIAN_POINT ( 'NONE',  ( 31.01321894478757812, -1.392741288986461212, -5.783357778048658027 ) ) ;
#4333=CARTESIAN_POINT ( 'NONE',  ( 31.49429780130001433, -5.496349022752856861, -7.939653947423664704 ) ) ;
#4346=CARTESIAN_POINT ( 'NONE',  ( 32.87199790123699472, -1.558343308739095656, -5.783357778048663356 ) ) ;
#4347=CARTESIAN_POINT ( 'NONE',  ( 28.75786045390062995, -2.691183018653962034, -6.861505862736159145 ) ) ;
#4350=ORIENTED_EDGE ( 'NONE', *, *, #2408, .F. ) ;
#4363=CARTESIAN_POINT ( 'NONE',  ( 29.62489513447700062, -6.348545659133139729, -6.861505862736166250 ) ) ;
#4366=AXIS2_PLACEMENT_3D ( 'NONE', #13163, #4633, #3372 ) ;
#4368=CARTESIAN_POINT ( 'NONE',  ( 38.64694918415791136, -1.054552983374777986, -9.783357778048662468 ) ) ;
#4380=CARTESIAN_POINT ( 'NONE',  ( 31.94023320572814484, -7.096308717197083560, -5.783357778048669573 ) ) ;
#4390=FILL_AREA_STYLE_COLOUR ( '', #11954 ) ;
#4401=CARTESIAN_POINT ( 'NONE',  ( 32.92264866086529906, -1.552240892477451339, -6.453230759126466154 ) ) ;
#4408=EDGE_CURVE ( 'NONE', #3520, #16322, #1090, .T. ) ;
#4409=ORIENTED_EDGE ( 'NONE', *, *, #11476, .F. ) ;
#4416=CARTESIAN_POINT ( 'NONE',  ( 38.02246887229409111, 4.128705714927905390, 0.2592325134722451851 ) ) ;
#4422=CARTESIAN_POINT ( 'NONE',  ( 33.17547354829333273, -5.293800545841212291, -3.627061608673667781 ) ) ;
#4426=CARTESIAN_POINT ( 'NONE',  ( 31.91006497951310550, -2.311404624444611589, -6.861505862736159145 ) ) ;
#4429=( BOUNDED_CURVE ( )  B_SPLINE_CURVE ( 2, ( #2790, #4658, #15819, #7478, #15637, #9742, #6955, #416, #5921 ),
 .UNSPECIFIED., .F., .T. ) 
 B_SPLINE_CURVE_WITH_KNOTS ( ( 3, 2, 2, 2, 3 ),
 ( 0.9038461538461538547, 0.9102564102564102422, 0.9230769230769231282, 0.9358974358974359031, 0.9423076923076922906 ),
 .UNSPECIFIED. ) 
 CURVE ( )  GEOMETRIC_REPRESENTATION_ITEM ( )  RATIONAL_B_SPLINE_CURVE ( ( 0.9330127018922194093, 0.9330127018922194093, 1.000000000000000000, 0.8660254037844387076, 1.000000000000000000, 0.8660254037844387076, 1.000000000000000000, 0.9330127018922194093, 0.9330127018922194093 ) ) 
 REPRESENTATION_ITEM ( '' )  );
#4431=CARTESIAN_POINT ( 'NONE',  ( 30.71189515440122975, -6.854751018602581958, -5.783357778048663356 ) ) ;
#4436=AXIS2_PLACEMENT_3D ( 'NONE', #4368, #14155, #12701 ) ;
#4441=CARTESIAN_POINT ( 'NONE',  ( 31.65190802758064592, -5.477360103042387074, -7.939653947423664704 ) ) ;
#4455=CARTESIAN_POINT ( 'NONE',  ( 25.99795558426325215, -4.648046406214923820, -3.627061608673664228 ) ) ;
#4466=LINE ( 'NONE', #14079, #567 ) ;
#4469=CARTESIAN_POINT ( 'NONE',  ( 32.33415724766913257, -1.960501102408027219, -4.533357778048659803 ) ) ;
#4486=DIRECTION ( 'NONE',  ( -0.9928203230275512992, -0.1196152422706610319, -9.614813431917826478E-17 ) ) ;
#4502=VERTEX_POINT ( 'NONE', #12950 ) ;
#4508=CARTESIAN_POINT ( 'NONE',  ( 27.57216386142120257, -6.895668018177890879, -7.033357778048666908 ) ) ;
#4511=CARTESIAN_POINT ( 'NONE',  ( 32.54503264317084188, -5.369756224683081669, -3.627061608673667781 ) ) ;
#4514=CARTESIAN_POINT ( 'NONE',  ( 27.38828526237195504, -6.917821758047558056, -4.533357778048668685 ) ) ;
#4523=DIRECTION ( 'NONE',  ( 0.9928203230275510771, 0.1196152422706609902, 4.006172263299092517E-17 ) ) ;
#4524=CARTESIAN_POINT ( 'NONE',  ( 31.44176105920648823, -5.502678662656354192, -3.627061608673668225 ) ) ;
#4536=CARTESIAN_POINT ( 'NONE',  ( 26.21417678486618641, -2.370676134166772808, -5.783357778048658915 ) ) ;
#4543=VECTOR ( 'NONE', #8436, 1000.000000000000227 ) ;
#4552=CARTESIAN_POINT ( 'NONE',  ( 32.92339180097568629, -5.524043937428110063, -3.283357778048667797 ) ) ;
#4556=EDGE_CURVE ( 'NONE', #10267, #15625, #16054, .T. ) ;
#4566=ORIENTED_EDGE ( 'NONE', *, *, #11072, .F. ) ;
#4575=FACE_OUTER_BOUND ( 'NONE', #9715, .T. ) ;
#4576=CARTESIAN_POINT ( 'NONE',  ( 46.37688276194213444, -2.449350377220338881, -5.783357778048662468 ) ) ;
#4580=CARTESIAN_POINT ( 'NONE',  ( 27.10313151398701947, -6.652368374500619908, -6.861505862736166250 ) ) ;
#4581=ORIENTED_EDGE ( 'NONE', *, *, #6190, .T. ) ;
#4584=CARTESIAN_POINT ( 'NONE',  ( 32.60321786976872005, -6.626883982076972934, -5.783357778048663356 ) ) ;
#4585=CYLINDRICAL_SURFACE ( 'NONE', #7601, 2.500000000000001776 ) ;
#4586=VERTEX_POINT ( 'NONE', #4211 ) ;
#4588=AXIS2_PLACEMENT_3D ( 'NONE', #17109, #3313, #11449 ) ;
#4594=CARTESIAN_POINT ( 'NONE',  ( 26.63392073224175505, -2.647267031729148012, -7.033357778048658027 ) ) ;
#4595=CARTESIAN_POINT ( 'NONE',  ( 32.52441275490655670, -6.636378442139655220, -5.783357778048663356 ) ) ;
#4597=CARTESIAN_POINT ( 'NONE',  ( 30.78070346053490880, -6.209293581256383199, -4.705209693361168455 ) ) ;
#4599=CARTESIAN_POINT ( 'NONE',  ( 26.19678349485696955, -4.880653813392439311, -3.627061608673664672 ) ) ;
#4612=CARTESIAN_POINT ( 'NONE',  ( 33.30663696749426350, -1.516174747195733863, -5.783357778048658027 ) ) ;
#4616=CARTESIAN_POINT ( 'NONE',  ( 27.50829672905005907, -3.268828784122926212, -3.283357778048662023 ) ) ;
#4618=B_SPLINE_CURVE_WITH_KNOTS ( 'NONE', 3,
 ( #3567, #16173, #7728, #10436, #17469, #2215, #11982, #3918, #12062, #17649, #5259, #9349, #13255, #14887, #14634, #6275, #14969, #17565 ),
 .UNSPECIFIED., .F., .F.,
 ( 4, 2, 2, 2, 2, 2, 2, 2, 4 ),
 ( 0.000000000000000000, 0.0005710890023745246154, 0.001142178004749049231, 0.001713267007123573955, 0.002284356009498098462, 0.002855445011872622969, 0.003426534014247147909, 0.003997623016621672416, 0.004568712018996196923 ),
 .UNSPECIFIED. ) ;
#4621=CARTESIAN_POINT ( 'NONE',  ( 30.66050125466253107, -2.889050389913576655, -3.283357778048662023 ) ) ;
#4627=CARTESIAN_POINT ( 'NONE',  ( 26.99805802979993885, -6.665027654307603022, -4.705209693361168455 ) ) ;
#4633=DIRECTION ( 'NONE',  ( 0.9928203230275511881, 0.1196152422706609764, 1.201851678989727817E-16 ) ) ;
#4638=CARTESIAN_POINT ( 'NONE',  ( 26.82912971812489644, -6.258282166232842947, -8.283357778048664244 ) ) ;
#4646=CARTESIAN_POINT ( 'NONE',  ( 30.40162818048570514, -5.827866652795590241, -3.283357778048667797 ) ) ;
#4658=CARTESIAN_POINT ( 'NONE',  ( 26.82229025357024454, -7.323371595517525812, -5.113484796970862334 ) ) ;
#4665=CARTESIAN_POINT ( 'NONE',  ( 33.33308377457396432, -5.274811626130743392, -3.627061608673668225 ) ) ;
#4667=EDGE_CURVE ( 'NONE', #7301, #9127, #15277, .T. ) ;
#4671=ORIENTED_EDGE ( 'NONE', *, *, #16092, .T. ) ;
#4676=DIRECTION ( 'NONE',  ( 0.9928203230275512992, 0.1196152422706610180, 4.006172263299093133E-17 ) ) ;
#4684=CARTESIAN_POINT ( 'NONE',  ( 28.16881664323205570, -6.096876348486420127, -8.283357778048662468 ) ) ;
#4687=CARTESIAN_POINT ( 'NONE',  ( 41.60261161686052134, -0.5064767720214736757, -5.783357778048662468 ) ) ;
#4689=CARTESIAN_POINT ( 'NONE',  ( 28.86293393808771057, -2.678523738846987357, -4.705209693361161349 ) ) ;
#4691=CARTESIAN_POINT ( 'NONE',  ( 25.77386970449396841, -2.888308184441632953, -6.623114134516397300 ) ) ;
#4696=AXIS2_PLACEMENT_3D ( 'NONE', #10834, #2700, #3884 ) ;
#4702=CARTESIAN_POINT ( 'NONE',  ( 32.67619606237177265, -1.592130426037603907, -5.783357778048658027 ) ) ;
#4704=CARTESIAN_POINT ( 'NONE',  ( 27.24868051476284236, -2.235842002054281075, -6.453230759126464378 ) ) ;
#4709=ORIENTED_EDGE ( 'NONE', *, *, #14626, .T. ) ;
#4710=ORIENTED_EDGE ( 'NONE', *, *, #1345, .F. ) ;
#4717=( BOUNDED_CURVE ( )  B_SPLINE_CURVE ( 2, ( #13140, #10748, #16058, #6334, #7700, #13319, #13226, #14607, #2093 ),
 .UNSPECIFIED., .F., .T. ) 
 B_SPLINE_CURVE_WITH_KNOTS ( ( 3, 2, 2, 2, 3 ),
 ( 0.4807692307692307820, 0.4871794871794871695, 0.5000000000000000000, 0.5128205128205127750, 0.5192307692307692735 ),
 .UNSPECIFIED. ) 
 CURVE ( )  GEOMETRIC_REPRESENTATION_ITEM ( )  RATIONAL_B_SPLINE_CURVE ( ( 0.9330127018922194093, 0.9330127018922196314, 1.000000000000000000, 0.8660254037844387076, 1.000000000000000000, 0.8660254037844387076, 1.000000000000000000, 0.9330127018922187432, 0.9330127018922192983 ) ) 
 REPRESENTATION_ITEM ( '' )  );
#4723=PLANE ( 'NONE',  #4366 ) ;
#4733=CARTESIAN_POINT ( 'NONE',  ( 29.27960797773944179, -6.689954721521948144, -4.533357778048668685 ) ) ;
#4740=FACE_OUTER_BOUND ( 'NONE', #10670, .T. ) ;
#4745=CARTESIAN_POINT ( 'NONE',  ( 25.76974524478944062, -2.854074692636065169, -5.141149657938114181 ) ) ;
#4746=CARTESIAN_POINT ( 'NONE',  ( 26.31065902414478330, -7.328232685206446106, -6.312034385895062272 ) ) ;
#4747=LINE ( 'NONE', #10272, #5571 ) ;
#4752=CARTESIAN_POINT ( 'NONE',  ( 28.30694982360322953, -3.372479377640031473, -7.939653947423660263 ) ) ;
#4757=VERTEX_POINT ( 'NONE', #14458 ) ;
#4758=CARTESIAN_POINT ( 'NONE',  ( 27.08121146544255353, -6.028038774645947839, -7.939653947423664704 ) ) ;
#4759=ORIENTED_EDGE ( 'NONE', *, *, #13089, .T. ) ;
#4766=ADVANCED_FACE ( 'NONE', ( #4740 ), #4821, .T. ) ;
#4771=CARTESIAN_POINT ( 'NONE',  ( 26.78782184427022983, -4.809445364374452581, -8.283357778048662468 ) ) ;
#4775=CARTESIAN_POINT ( 'NONE',  ( 29.39282811755836633, -5.749534618892433002, -3.627061608673667781 ) ) ;
#4779=ORIENTED_EDGE ( 'NONE', *, *, #2478, .F. ) ;
#4781=ORIENTED_EDGE ( 'NONE', *, *, #9449, .T. ) ;
#4790=CARTESIAN_POINT ( 'NONE',  ( 31.54230778485832332, -2.355712103769039611, -4.705209693361160461 ) ) ;
#4793=CARTESIAN_POINT ( 'NONE',  ( 26.73899421642883567, -2.634607751922174224, -4.533357778048659803 ) ) ;
#4799=LINE ( 'NONE', #6448, #14434 ) ;
#4806=EDGE_CURVE ( 'NONE', #13578, #13615, #10338, .T. ) ;
#4809=VERTEX_POINT ( 'NONE', #580 ) ;
#4810=CARTESIAN_POINT ( 'NONE',  ( 30.01512236704901682, -6.601339762873093875, -7.033357778048666908 ) ) ;
#4813=DIRECTION ( 'NONE',  ( -0.9928203230275511881, -0.1196152422706610041, -4.006172263299093133E-17 ) ) ;
#4816=CARTESIAN_POINT ( 'NONE',  ( 27.52714686987067694, -7.627998469090175426, -5.783357778048669573 ) ) ;
#4817=CARTESIAN_POINT ( 'NONE',  ( 31.75254397038802878, -4.211294393702175398, -8.283357778048662468 ) ) ;
#4820=VERTEX_POINT ( 'NONE', #4916 ) ;
#4821=CYLINDRICAL_SURFACE ( 'NONE', #5703, 2.500000000000001776 ) ;
#4838=CARTESIAN_POINT ( 'NONE',  ( 29.78250536075762867, -6.329556739422670830, -6.861505862736167138 ) ) ;
#4844=ORIENTED_EDGE ( 'NONE', *, *, #6121, .F. ) ;
#4851=ORIENTED_EDGE ( 'NONE', *, *, #4267, .F. ) ;
#4856=CARTESIAN_POINT ( 'NONE',  ( 30.67110321781257909, -3.087645581983020637, -7.939653947423660263 ) ) ;
#4862=CARTESIAN_POINT ( 'NONE',  ( 26.21417678486618641, -2.370676134166772808, -5.783357778048658027 ) ) ;
#4867=ORIENTED_EDGE ( 'NONE', *, *, #12700, .T. ) ;
#4869=AXIS2_PLACEMENT_3D ( 'NONE', #14029, #7147, #15291 ) ;
#4876=LINE ( 'NONE', #6431, #9811 ) ;
#4878=CARTESIAN_POINT ( 'NONE',  ( 27.77288575766320378, -4.690764616287755651, -7.939653947423662039 ) ) ;
#4880=CARTESIAN_POINT ( 'NONE',  ( 27.26436163736424945, -2.571311352887278190, -7.033357778048658027 ) ) ;
#4882=DIRECTION ( 'NONE',  ( -0.6951637808321682321, 0.2969442527608448512, 0.6546536707079773088 ) ) ;
#4885=ORIENTED_EDGE ( 'NONE', *, *, #17671, .T. ) ;
#4887=CARTESIAN_POINT ( 'NONE',  ( 31.87075164095941915, -4.197052703815608687, -3.627061608673664672 ) ) ;
#4889=DIRECTION ( 'NONE',  ( 0.9928203230275512992, 0.1196152422706610180, 4.006172263299093133E-17 ) ) ;
#4911=CARTESIAN_POINT ( 'NONE',  ( 28.05993251931039012, -3.202367565343739564, -3.283357778048662023 ) ) ;
#4913=CARTESIAN_POINT ( 'NONE',  ( 31.71314141467879111, -4.216041623526076698, -3.627061608673664672 ) ) ;
#4916=CARTESIAN_POINT ( 'NONE',  ( 38.62415064777786000, -0.8653224988334575762, -5.783357778048662468 ) ) ;
#4922=CARTESIAN_POINT ( 'NONE',  ( 25.78162057792670225, -2.952641328940847743, -4.882123357130833341 ) ) ;
#4928=LINE ( 'NONE', #14905, #3978 ) ;
#4929=CARTESIAN_POINT ( 'NONE',  ( 31.24031073583692475, -4.273008382657478954, -3.627061608673664672 ) ) ;
#4934=EDGE_CURVE ( 'NONE', #9123, #7189, #5008, .T. ) ;
#4936=DIRECTION ( 'NONE',  ( -0.9569661826241284697, -0.2901994578110082545, -1.159531966109436593E-16 ) ) ;
#4949=CARTESIAN_POINT ( 'NONE',  ( 31.88814493096863956, -1.687075024589942851, -5.783357778048658027 ) ) ;
#4952=CARTESIAN_POINT ( 'NONE',  ( 28.35948656569675919, -3.366149737736551906, -3.627061608673662896 ) ) ;
#4962=VECTOR ( 'NONE', #2640, 1000.000000000000227 ) ;
#4967=ORIENTED_EDGE ( 'NONE', *, *, #12198, .F. ) ;
#4970=CARTESIAN_POINT ( 'NONE',  ( 29.04699097144805364, -6.418171698071525100, -4.705209693361169343 ) ) ;
#4982=CARTESIAN_POINT ( 'NONE',  ( 30.78487334700428235, -1.819997462563214263, -5.783357778048658915 ) ) ;
#4995=CARTESIAN_POINT ( 'NONE',  ( 29.71979337562451207, -1.938121702948446323, -5.783357778048664244 ) ) ;
#5004=CARTESIAN_POINT ( 'NONE',  ( 28.48022645605872327, -3.151730446115816875, -8.283357778048658915 ) ) ;
#5008=LINE ( 'NONE', #12412, #10641 ) ;
#5009=CARTESIAN_POINT ( 'NONE',  ( 29.79859849048667897, -1.928627242885762705, -5.783357778048664244 ) ) ;
#5013=CARTESIAN_POINT ( 'NONE',  ( 33.68284756902015431, -1.652629194728084450, -1.783357778048662912 ) ) ;
#5024=CARTESIAN_POINT ( 'NONE',  ( 29.65098506949083301, -2.583579140294649523, -4.705209693361160461 ) ) ;
#5028=ORIENTED_EDGE ( 'NONE', *, *, #13273, .T. ) ;
#5040=CARTESIAN_POINT ( 'NONE',  ( 30.62726312072365431, -1.838986382273682718, -5.783357778048658027 ) ) ;
#5044=CARTESIAN_POINT ( 'NONE',  ( 29.62489513447700062, -6.348545659133139729, -6.861505862736166250 ) ) ;
#5058=CARTESIAN_POINT ( 'NONE',  ( 29.17398450417959310, -7.029842018119214941, -5.783357778048669573 ) ) ;
#5060=CARTESIAN_POINT ( 'NONE',  ( 32.01903832059031174, -7.086814257134402162, -5.783357778048669573 ) ) ;
#5067=CARTESIAN_POINT ( 'NONE',  ( 32.17274868998081416, -2.279756424927169345, -4.705209693361160461 ) ) ;
#5068=ORIENTED_EDGE ( 'NONE', *, *, #3627, .T. ) ;
#5069=EDGE_CURVE ( 'NONE', #7075, #15926, #17188, .T. ) ;
#5071=CARTESIAN_POINT ( 'NONE',  ( 34.23532670761333918, -6.238269840783186027, -9.783357778048662468 ) ) ;
#5082=ORIENTED_EDGE ( 'NONE', *, *, #13089, .F. ) ;
#5088=CARTESIAN_POINT ( 'NONE',  ( 29.98133424373737910, -5.878503772023492502, -8.283357778048662468 ) ) ;
#5089=CARTESIAN_POINT ( 'NONE',  ( 31.41114436565740320, -6.133337902414513820, -4.705209693361168455 ) ) ;
#5090=ADVANCED_FACE ( 'NONE', ( #7434 ), #14130, .T. ) ;
#5091=ORIENTED_EDGE ( 'NONE', *, *, #6986, .F. ) ;
#5095=CARTESIAN_POINT ( 'NONE',  ( 0.000000000000000000, 0.000000000000000000, 0.000000000000000000 ) ) ;
#5105=CARTESIAN_POINT ( 'NONE',  ( 29.54591158530375239, -2.596238420101622868, -6.861505862736158257 ) ) ;
#5106=CARTESIAN_POINT ( 'NONE',  ( 33.40754056521197413, -5.892811586081919906, -6.861505862736166250 ) ) ;
#5121=CARTESIAN_POINT ( 'NONE',  ( 30.75425665345519732, -2.450656702321377001, -4.705209693361161349 ) ) ;
#5129=CARTESIAN_POINT ( 'NONE',  ( 47.10521669518294630, -4.378041487036774981, -5.783357778048661579 ) ) ;
#5140=CARTESIAN_POINT ( 'NONE',  ( 30.06013935859953534, -5.869009311960809328, -8.283357778048664244 ) ) ;
#5142=CARTESIAN_POINT ( 'NONE',  ( 28.28502977505876359, -2.748149777785362957, -6.861505862736158257 ) ) ;
#5150=CARTESIAN_POINT ( 'NONE',  ( 30.81132015408399027, -5.578634341498224458, -3.627061608673668225 ) ) ;
#5152=( BOUNDED_CURVE ( )  B_SPLINE_CURVE ( 2, ( #13070, #655, #6177, #15887, #2119, #12892, #3462, #6266, #476 ),
 .UNSPECIFIED., .F., .T. ) 
 B_SPLINE_CURVE_WITH_KNOTS ( ( 3, 2, 2, 2, 3 ),
 ( 0.5192307692307692735, 0.5256410256410256610, 0.5384615384615384359, 0.5512820512820513219, 0.5576923076923077094 ),
 .UNSPECIFIED. ) 
 CURVE ( )  GEOMETRIC_REPRESENTATION_ITEM ( )  RATIONAL_B_SPLINE_CURVE ( ( 0.9330127018922192983, 0.9330127018922198534, 1.000000000000000000, 0.8660254037844387076, 1.000000000000000000, 0.8660254037844387076, 1.000000000000000000, 0.9330127018922194093, 0.9330127018922194093 ) ) 
 REPRESENTATION_ITEM ( '' )  );
#5161=CARTESIAN_POINT ( 'NONE',  ( 26.04410741498555382, -2.380969272135942560, -5.113484796970857893 ) ) ;
#5167=ORIENTED_EDGE ( 'NONE', *, *, #1129, .F. ) ;
#5174=CARTESIAN_POINT ( 'NONE',  ( 26.18945719470476163, -6.341381504099093291, -7.820351782355674963 ) ) ;
#5175=CARTESIAN_POINT ( 'NONE',  ( 33.60446413004628141, -3.988174587000466342, -3.627061608673664672 ) ) ;
#5192=CARTESIAN_POINT ( 'NONE',  ( 27.14244485254070938, -4.766720295129625029, -7.939653947423662039 ) ) ;
#5193=CARTESIAN_POINT ( 'NONE',  ( 25.92467471225709374, -2.732717170633701453, -7.033357778048658027 ) ) ;
#5196=ORIENTED_EDGE ( 'NONE', *, *, #4091, .F. ) ;
#5205=LINE ( 'NONE', #16125, #1535 ) ;
#5208=ORIENTED_EDGE ( 'NONE', *, *, #4556, .T. ) ;
#5226=AXIS2_PLACEMENT_3D ( 'NONE', #17157, #7528, #3267 ) ;
#5229=CARTESIAN_POINT ( 'NONE',  ( 29.77797860222238313, -3.195249460342344250, -3.627061608673662008 ) ) ;
#5231=CARTESIAN_POINT ( 'NONE',  ( 33.04340326765378677, -1.875050963503474222, -4.533357778048659803 ) ) ;
#5240=CARTESIAN_POINT ( 'NONE',  ( 32.93470988637010066, -5.949778345213319497, -6.861505862736167138 ) ) ;
#5244=ORIENTED_EDGE ( 'NONE', *, *, #15743, .F. ) ;
#5250=CARTESIAN_POINT ( 'NONE',  ( 26.83664947211162399, -6.984282976826746037, -4.533357778048668685 ) ) ;
#5259=CARTESIAN_POINT ( 'NONE',  ( 26.24651417059167358, -6.811311830135031720, -4.396611942026659392 ) ) ;
#5264=CARTESIAN_POINT ( 'NONE',  ( 33.14902674121363901, -1.535163666906202318, -5.783357778048658915 ) ) ;
#5265=EDGE_CURVE ( 'NONE', #9127, #13220, #1997, .T. ) ;
#5274=VECTOR ( 'NONE', #14997, 1000.000000000000227 ) ;
#5278=( BOUNDED_SURFACE ( )  B_SPLINE_SURFACE ( 1, 2, ( 
 ( #5930, #14193, #17021, #11644, #11454, #8568, #14294, #17212, #11362, #14019, #12918, #4665, #11258, #1881, #10193, #8845, #15465, #6017, #1688, #7408, #503, #3048, #10096, #7223, #7485, #12735, #332, #3318, #15645, #1603, #16932, #10004, #17113, #9821, #3131, #14381, #15371, #2954, #17399, #14654, #17499, #3762, #7579, #771, #15918, #12004, #13107, #2237, #4929, #7749, #10624, #11728, #14741, #2328, #16197, #9284, #14825, #9116, #13471, #10364, #685, #860, #3493, #13280, #2151, #2057, #9196, #6299, #6393, #12084, #15827, #6211, #17300, #11910, #5024, #7670, #5105, #7847, #13194, #10546, #4838, #3400, #10461, #7934, #2413, #1044, #16110, #10278, #3671, #14574, #13373, #8930, #11820, #6564, #14473, #16022, #956, #9024, #3593, #6489, #17585, #4752, #12356, #17757, #2835, #3855, #16629, #15176, #6650, #6831, #2757, #4206, #17924, #12180, #8276, #9538, #13636, #13807, #1125, #3937, #5365, #9624, #1394, #11068, #5456, #10975, #5192, #6915, #15085, #5282, #1488, #8363, #12448, #10712, #8011, #10799, #16537, #35, #7016, #5544, #9706, #4115, #13894, #1309, #10885, #15256, #16454, #16374, #14906, #8102, #1226, #2668, #8198, #17669, #16285 ),
 ( #17846, #13724, #9366, #9452, #2489, #13550, #14989, #2575, #6741, #4022, #12277, #212, #2929, #8640, #5720, #15529, #9893, #9798, #16998, #14081, #305, #16718, #8550, #4552, #14360, #16815, #4469, #3111, #1581, #10074, #15349, #5996, #15621, #14170, #3199, #11238, #8740, #1945, #16913, #15445, #403, #8828, #8464, #11434, #123, #4380, #12540, #3026, #11337, #1667, #7115, #7203, #13997, #12628, #7388, #9982, #1760, #12712, #5815, #1859, #7291, #10172, #12809, #5632, #11148, #5909, #14270, #12902, #486, #11523, #17091, #4646, #15723, #3298, #4289, #6093, #7652, #10609, #17568, #5088, #17377, #12989, #9095, #17280, #7731, #11622, #10345, #9263, #17187, #2131, #10439, #3381, #8914, #2218, #4733, #16176, #13258, #7557, #3738, #10257, #6471, #5004, #14451, #14637, #10529, #11985, #840, #2032, #16090, #4911, #3472, #3657, #13083, #11709, #13175, #17473, #9178, #934, #6369, #11892, #574, #14722, #15999, #664, #14808, #7465, #2306, #15807, #6187, #4816, #7824, #13355, #15898, #9002, #14550, #751, #6278, #11799, #3572, #17908, #8086, #9352, #17651, #10782, #16360, #5347, #17828, #1294, #15159, #10689, #10868, #14890, #5174, #6633, #2476 ) ),
 .UNSPECIFIED., .F., .F., .T. ) 
 B_SPLINE_SURFACE_WITH_KNOTS ( ( 2, 2 ),
 ( 3, 2, 2, 2, 2, 2, 2, 2, 2, 2, 2, 2, 2, 2, 2, 2, 2, 2, 2, 2, 2, 2, 2, 2, 2, 2, 2, 2, 2, 2, 2, 2, 2, 2, 2, 2, 2, 2, 2, 2, 2, 2, 2, 2, 2, 2, 2, 2, 2, 2, 2, 2, 2, 2, 2, 2, 2, 2, 2, 2, 2, 2, 2, 2, 2, 2, 2, 2, 2, 2, 2, 2, 2, 2, 2, 2, 2, 3 ),
 ( 0.000000000000000000, 1.000000000000000000 ),
 ( 0.000000000000000000, 0.01282051282051282007, 0.02564102564102564014, 0.03846153846153846367, 0.05128205128205128027, 0.06410256410256409687, 0.07692307692307692735, 0.08974358974358974395, 0.1025641025641025605, 0.1153846153846153910, 0.1282051282051281937, 0.1410256410256410242, 0.1538461538461538547, 0.1666666666666666574, 0.1794871794871794879, 0.1923076923076923184, 0.2051282051282051211, 0.2179487179487179516, 0.2307692307692307820, 0.2435897435897435848, 0.2564102564102563875, 0.2692307692307692180, 0.2820512820512820484, 0.2948717948717948789, 0.3076923076923077094, 0.3205128205128205399, 0.3333333333333333148, 0.3461538461538461453, 0.3589743589743589758, 0.3717948717948718063, 0.3846153846153846367, 0.3974358974358974117, 0.4102564102564102422, 0.4230769230769230727, 0.4358974358974359031, 0.4487179487179487336, 0.4615384615384615641, 0.4743589743589743390, 0.4871794871794871695, 0.5000000000000000000, 0.5128205128205127750, 0.5256410256410256610, 0.5384615384615384359, 0.5512820512820513219, 0.5641025641025640969, 0.5769230769230768718, 0.5897435897435897578, 0.6025641025641025328, 0.6153846153846154188, 0.6282051282051281937, 0.6410256410256410797, 0.6538461538461538547, 0.6666666666666666297, 0.6794871794871795156, 0.6923076923076922906, 0.7051282051282051766, 0.7179487179487179516, 0.7307692307692307265, 0.7435897435897436125, 0.7564102564102563875, 0.7692307692307692735, 0.7820512820512820484, 0.7948717948717948234, 0.8076923076923077094, 0.8205128205128204844, 0.8333333333333333703, 0.8461538461538461453, 0.8589743589743589203, 0.8717948717948718063, 0.8846153846153845812, 0.8974358974358974672, 0.9102564102564102422, 0.9230769230769231282, 0.9358974358974359031, 0.9487179487179486781, 0.9615384615384615641, 0.9690837477411259338, 0.9787745852185372186 ),
 .UNSPECIFIED. ) 
 GEOMETRIC_REPRESENTATION_ITEM ( )  RATIONAL_B_SPLINE_SURFACE ( (
 ( 1.000000000000000000, 0.8660254037844387076, 1.000000000000000000, 0.8660254037844387076, 1.000000000000000000, 0.8660254037844387076, 1.000000000000000000, 0.8660254037844387076, 1.000000000000000000, 0.8660254037844387076, 1.000000000000000000, 0.8660254037844387076, 1.000000000000000000, 0.8660254037844387076, 1.000000000000000000, 0.8660254037844387076, 1.000000000000000000, 0.8660254037844387076, 1.000000000000000000, 0.8660254037844387076, 1.000000000000000000, 0.8660254037844387076, 1.000000000000000000, 0.8660254037844387076, 1.000000000000000000, 0.8660254037844387076, 1.000000000000000000, 0.8660254037844387076, 1.000000000000000000, 0.8660254037844387076, 1.000000000000000000, 0.8660254037844387076, 1.000000000000000000, 0.8660254037844387076, 1.000000000000000000, 0.8660254037844387076, 1.000000000000000000, 0.8660254037844387076, 1.000000000000000000, 0.8660254037844387076, 1.000000000000000000, 0.8660254037844387076, 1.000000000000000000, 0.8660254037844387076, 1.000000000000000000, 0.8660254037844387076, 1.000000000000000000, 0.8660254037844387076, 1.000000000000000000, 0.8660254037844387076, 1.000000000000000000, 0.8660254037844387076, 1.000000000000000000, 0.8660254037844387076, 1.000000000000000000, 0.8660254037844387076, 1.000000000000000000, 0.8660254037844387076, 1.000000000000000000, 0.8660254037844387076, 1.000000000000000000, 0.8660254037844387076, 1.000000000000000000, 0.8660254037844387076, 1.000000000000000000, 0.8660254037844387076, 1.000000000000000000, 0.8660254037844387076, 1.000000000000000000, 0.8660254037844387076, 1.000000000000000000, 0.8660254037844387076, 1.000000000000000000, 0.8660254037844387076, 1.000000000000000000, 0.8660254037844387076, 1.000000000000000000, 0.8660254037844387076, 1.000000000000000000, 0.8660254037844387076, 1.000000000000000000, 0.8660254037844387076, 1.000000000000000000, 0.8660254037844387076, 1.000000000000000000, 0.8660254037844387076, 1.000000000000000000, 0.8660254037844387076, 1.000000000000000000, 0.8660254037844387076, 1.000000000000000000, 0.8660254037844387076, 1.000000000000000000, 0.8660254037844387076, 1.000000000000000000, 0.8660254037844387076, 1.000000000000000000, 0.8660254037844387076, 1.000000000000000000, 0.8660254037844387076, 1.000000000000000000, 0.8660254037844387076, 1.000000000000000000, 0.8660254037844387076, 1.000000000000000000, 0.8660254037844387076, 1.000000000000000000, 0.8660254037844387076, 1.000000000000000000, 0.8660254037844387076, 1.000000000000000000, 0.8660254037844387076, 1.000000000000000000, 0.8660254037844387076, 1.000000000000000000, 0.8660254037844387076, 1.000000000000000000, 0.8660254037844387076, 1.000000000000000000, 0.8660254037844387076, 1.000000000000000000, 0.8660254037844387076, 1.000000000000000000, 0.8660254037844387076, 1.000000000000000000, 0.8660254037844387076, 1.000000000000000000, 0.8660254037844387076, 1.000000000000000000, 0.8660254037844387076, 1.000000000000000000, 0.8660254037844387076, 1.000000000000000000, 0.8660254037844387076, 1.000000000000000000, 0.8660254037844387076, 1.000000000000000000, 0.8660254037844387076, 1.000000000000000000, 0.8660254037844387076, 1.000000000000000000, 0.8660254037844387076, 1.000000000000000000, 0.8660254037844387076, 1.000000000000000000, 0.8660254037844387076, 1.000000000000000000, 0.8660254037844387076, 1.000000000000000000, 0.8660254037844387076, 1.000000000000000000, 0.9211516195580409239, 0.9351128802560608744, 0.9351128802560608744, 0.9351128802560608744),
 ( 1.000000000000000000, 0.8660254037844387076, 1.000000000000000000, 0.8660254037844387076, 1.000000000000000000, 0.8660254037844387076, 1.000000000000000000, 0.8660254037844387076, 1.000000000000000000, 0.8660254037844387076, 1.000000000000000000, 0.8660254037844387076, 1.000000000000000000, 0.8660254037844387076, 1.000000000000000000, 0.8660254037844387076, 1.000000000000000000, 0.8660254037844387076, 1.000000000000000000, 0.8660254037844387076, 1.000000000000000000, 0.8660254037844387076, 1.000000000000000000, 0.8660254037844387076, 1.000000000000000000, 0.8660254037844387076, 1.000000000000000000, 0.8660254037844387076, 1.000000000000000000, 0.8660254037844387076, 1.000000000000000000, 0.8660254037844387076, 1.000000000000000000, 0.8660254037844387076, 1.000000000000000000, 0.8660254037844387076, 1.000000000000000000, 0.8660254037844387076, 1.000000000000000000, 0.8660254037844387076, 1.000000000000000000, 0.8660254037844387076, 1.000000000000000000, 0.8660254037844387076, 1.000000000000000000, 0.8660254037844387076, 1.000000000000000000, 0.8660254037844387076, 1.000000000000000000, 0.8660254037844387076, 1.000000000000000000, 0.8660254037844387076, 1.000000000000000000, 0.8660254037844387076, 1.000000000000000000, 0.8660254037844387076, 1.000000000000000000, 0.8660254037844387076, 1.000000000000000000, 0.8660254037844387076, 1.000000000000000000, 0.8660254037844387076, 1.000000000000000000, 0.8660254037844387076, 1.000000000000000000, 0.8660254037844387076, 1.000000000000000000, 0.8660254037844387076, 1.000000000000000000, 0.8660254037844387076, 1.000000000000000000, 0.8660254037844387076, 1.000000000000000000, 0.8660254037844387076, 1.000000000000000000, 0.8660254037844387076, 1.000000000000000000, 0.8660254037844387076, 1.000000000000000000, 0.8660254037844387076, 1.000000000000000000, 0.8660254037844387076, 1.000000000000000000, 0.8660254037844387076, 1.000000000000000000, 0.8660254037844387076, 1.000000000000000000, 0.8660254037844387076, 1.000000000000000000, 0.8660254037844387076, 1.000000000000000000, 0.8660254037844387076, 1.000000000000000000, 0.8660254037844387076, 1.000000000000000000, 0.8660254037844387076, 1.000000000000000000, 0.8660254037844387076, 1.000000000000000000, 0.8660254037844387076, 1.000000000000000000, 0.8660254037844387076, 1.000000000000000000, 0.8660254037844387076, 1.000000000000000000, 0.8660254037844387076, 1.000000000000000000, 0.8660254037844387076, 1.000000000000000000, 0.8660254037844387076, 1.000000000000000000, 0.8660254037844387076, 1.000000000000000000, 0.8660254037844387076, 1.000000000000000000, 0.8660254037844387076, 1.000000000000000000, 0.8660254037844387076, 1.000000000000000000, 0.8660254037844387076, 1.000000000000000000, 0.8660254037844387076, 1.000000000000000000, 0.8660254037844387076, 1.000000000000000000, 0.8660254037844387076, 1.000000000000000000, 0.8660254037844387076, 1.000000000000000000, 0.8660254037844387076, 1.000000000000000000, 0.8660254037844387076, 1.000000000000000000, 0.8660254037844387076, 1.000000000000000000, 0.8660254037844387076, 1.000000000000000000, 0.8660254037844387076, 1.000000000000000000, 0.8660254037844387076, 1.000000000000000000, 0.8660254037844387076, 1.000000000000000000, 0.8660254037844387076, 1.000000000000000000, 0.8660254037844387076, 1.000000000000000000, 0.8660254037844387076, 1.000000000000000000, 0.8660254037844387076, 1.000000000000000000, 0.9211516195580409239, 0.9351128802560608744, 0.9351128802560608744, 0.9351128802560608744) ) ) 
 REPRESENTATION_ITEM ( '' )  SURFACE ( )  );
#5282=CARTESIAN_POINT ( 'NONE',  ( 27.28266178881210280, -7.257709054644824853, -5.783357778048669573 ) ) ;
#5288=LINE ( 'NONE', #8109, #7548 ) ;
#5290=VERTEX_POINT ( 'NONE', #8880 ) ;
#5292=LINE ( 'NONE', #10811, #3182 ) ;
#5297=CARTESIAN_POINT ( 'NONE',  ( 25.71748644841968456, -2.420320648352046078, -5.783357778048663356 ) ) ;
#5319=LINE ( 'NONE', #3806, #12197 ) ;
#5325=CARTESIAN_POINT ( 'NONE',  ( 29.77797860222238313, -3.195249460342344250, -3.627061608673662008 ) ) ;
#5327=CARTESIAN_POINT ( 'NONE',  ( 33.40745134805642635, -4.011910736534825439, -3.283357778048664688 ) ) ;
#5338=UNCERTAINTY_MEASURE_WITH_UNIT (LENGTH_MEASURE( 1.000000000000000082E-05 ), #12550, 'distance_accuracy_value', 'NONE');
#5347=CARTESIAN_POINT ( 'NONE',  ( 26.16860980394290692, -3.430234601869349920, -3.283357778048662023 ) ) ;
#5348=CARTESIAN_POINT ( 'NONE',  ( 29.19137779418881351, -4.519864338893556877, -3.627061608673664672 ) ) ;
#5353=ORIENTED_EDGE ( 'NONE', *, *, #12316, .T. ) ;
#5365=CARTESIAN_POINT ( 'NONE',  ( 27.45766530510195835, -4.728742455708699666, -3.627061608673664672 ) ) ;
#5369=ADVANCED_FACE ( 'NONE', ( #14857 ), #13500, .T. ) ;
#5373=ORIENTED_EDGE ( 'NONE', *, *, #17531, .F. ) ;
#5378=ORIENTED_EDGE ( 'NONE', *, *, #15431, .T. ) ;
#5382=PRODUCT_DEFINITION_CONTEXT ( 'detailed design', #4243, 'design' ) ;
#5388=FACE_OUTER_BOUND ( 'NONE', #9335, .T. ) ;
#5396=ORIENTED_EDGE ( 'NONE', *, *, #10977, .F. ) ;
#5399=CARTESIAN_POINT ( 'NONE',  ( 31.00199007654869732, -2.847907730748336697, -8.283357778048660691 ) ) ;
#5402=CARTESIAN_POINT ( 'NONE',  ( 25.99533317148741318, -3.650983533393564517, -3.627061608673662008 ) ) ;
#5406=CARTESIAN_POINT ( 'NONE',  ( 30.03006034954003667, -2.965006068755446478, -3.283357778048662023 ) ) ;
#5407=CARTESIAN_POINT ( 'NONE',  ( 26.01652455409633902, -4.902371455920926380, -5.783357778048663356 ) ) ;
#5415=CARTESIAN_POINT ( 'NONE',  ( 28.54354359905709160, -7.105797696961086096, -5.783357778048669573 ) ) ;
#5421=EDGE_CURVE ( 'NONE', #2657, #8339, #3526, .T. ) ;
#5426=LINE ( 'NONE', #10943, #16252 ) ;
#5427=CARTESIAN_POINT ( 'NONE',  ( 28.36401332423200827, -6.500457016816879374, -6.861505862736166250 ) ) ;
#5428=CARTESIAN_POINT ( 'NONE',  ( 26.31556265977298992, -7.384422263489805793, -5.783357778048663356 ) ) ;
#5430=FACE_OUTER_BOUND ( 'NONE', #10125, .T. ) ;
#5441=CARTESIAN_POINT ( 'NONE',  ( 28.14933959732260149, -3.391468297350500372, -7.939653947423660263 ) ) ;
#5447=ORIENTED_EDGE ( 'NONE', *, *, #9395, .F. ) ;
#5456=CARTESIAN_POINT ( 'NONE',  ( 27.02414796481377124, -2.900061135469103490, -6.861505862736158257 ) ) ;
#5462=ORIENTED_EDGE ( 'NONE', *, *, #9447, .T. ) ;
#5489=CARTESIAN_POINT ( 'NONE',  ( 30.98067518586950442, -1.786210345264705790, -5.783357778048658027 ) ) ;
#5492=CARTESIAN_POINT ( 'NONE',  ( 27.02414796481377124, -2.900061135469103490, -6.861505862736158257 ) ) ;
#5495=CARTESIAN_POINT ( 'NONE',  ( 29.98885399772409954, -6.604504582617394703, -4.533357778048668685 ) ) ;
#5500=EDGE_CURVE ( 'NONE', #13220, #8853, #13564, .T. ) ;
#5503=CARTESIAN_POINT ( 'NONE',  ( 28.51709679197738723, -3.347160818026084339, -3.627061608673662008 ) ) ;
#5506=FACE_OUTER_BOUND ( 'NONE', #10442, .T. ) ;
#5517=CARTESIAN_POINT ( 'NONE',  ( 27.51889869220010354, -3.467423976192371082, -7.939653947423660263 ) ) ;
#5521=CIRCLE ( 'NONE', #7857, 1.000000000000000000 ) ;
#5529=CARTESIAN_POINT ( 'NONE',  ( 27.71165237056504793, -5.952083095804076684, -7.939653947423662927 ) ) ;
#5532=CARTESIAN_POINT ( 'NONE',  ( 39.16489837658902928, -5.353591089051432661, -9.283357778048653586 ) ) ;
#5544=CARTESIAN_POINT ( 'NONE',  ( 26.60838078660069428, -6.085005533777348319, -7.939653947423664704 ) ) ;
#5548=CIRCLE ( 'NONE', #16325, 2.500000000000001776 ) ;
#5549=ADVANCED_FACE ( 'NONE', ( #9737 ), #3061, .T. ) ;
#5551=DIRECTION ( 'NONE',  ( 0.05980762113533058533, -0.4964101615137755386, -0.8660254037844385966 ) ) ;
#5555=CARTESIAN_POINT ( 'NONE',  ( 28.53771668024168662, -2.080538600569502794, -5.783357778048658027 ) ) ;
#5556=ORIENTED_EDGE ( 'NONE', *, *, #12099, .T. ) ;
#5569=CARTESIAN_POINT ( 'NONE',  ( 26.01652455409633902, -4.902371455920926380, -5.783357778048663356 ) ) ;
#5571=VECTOR ( 'NONE', #15820, 1000.000000000000114 ) ;
#5584=CARTESIAN_POINT ( 'NONE',  ( 26.62577407660990758, -3.575027854551694695, -3.627061608673662008 ) ) ;
#5586=CARTESIAN_POINT ( 'NONE',  ( 28.49145532429760053, -1.696564004353941613, -5.783357778048658027 ) ) ;
#5587=CARTESIAN_POINT ( 'NONE',  ( 32.43181250335191379, -6.310176327312596811, -4.533357778048668685 ) ) ;
#5588=DIRECTION ( 'NONE',  ( 0.9928203230275512992, 0.1196152422706607682, -0.000000000000000000 ) ) ;
#5590=CARTESIAN_POINT ( 'NONE',  ( 29.49337484321020497, -2.602568060005117090, -4.705209693361161349 ) ) ;
#5591=CARTESIAN_POINT ( 'NONE',  ( 27.67650891848073158, -3.448435056481901295, -7.939653947423660263 ) ) ;
#5592=EDGE_LOOP ( 'NONE', ( #15951, #15562, #4867, #8977 ) ) ;
#5601=CARTESIAN_POINT ( 'NONE',  ( 32.95080301609915097, -1.548848848676412482, -5.783357778048662468 ) ) ;
#5603=CARTESIAN_POINT ( 'NONE',  ( 30.02326902268086428, -5.673578940050561847, -3.627061608673667781 ) ) ;
#5605=CARTESIAN_POINT ( 'NONE',  ( 37.11592063525292673, -0.6724158536360932414, -10.75768461118259545 ) ) ;
#5607=DIRECTION ( 'NONE',  ( -0.1196152422706610735, 0.9928203230275511881, 0.000000000000000000 ) ) ;
#5615=CARTESIAN_POINT ( 'NONE',  ( 28.24571643650507369, -4.633797857156355171, -7.939653947423662039 ) ) ;
#5631=ORIENTED_EDGE ( 'NONE', *, *, #1305, .T. ) ;
#5632=CARTESIAN_POINT ( 'NONE',  ( 30.30397292480292037, -1.478191427891014431, -5.783357778048658027 ) ) ;
#5651=CYLINDRICAL_SURFACE ( 'NONE', #4588, 2.500000000000001776 ) ;
#5658=DIRECTION ( 'NONE',  ( -0.1196152422706610735, 0.9928203230275511881, 0.000000000000000000 ) ) ;
#5663=CARTESIAN_POINT ( 'NONE',  ( 31.74131510559286085, -5.666460835049167422, -3.283357778048667797 ) ) ;
#5672=CARTESIAN_POINT ( 'NONE',  ( 27.91310269393460430, -7.181753375802955475, -5.783357778048669573 ) ) ;
#5674=CARTESIAN_POINT ( 'NONE',  ( 30.38277803966508372, -1.468696967828331701, -5.783357778048658027 ) ) ;
#5677=CARTESIAN_POINT ( 'NONE',  ( 31.08270050955629671, -4.291997302367946077, -3.627061608673664672 ) ) ;
#5679=EDGE_CURVE ( 'NONE', #7873, #1701, #2078, .T. ) ;
#5691=CARTESIAN_POINT ( 'NONE',  ( 28.86293393808771057, -2.678523738846987357, -4.705209693361161349 ) ) ;
#5693=CARTESIAN_POINT ( 'NONE',  ( 26.31556265977298992, -7.384422263489805793, -5.783357778048663356 ) ) ;
#5694=CARTESIAN_POINT ( 'NONE',  ( 27.30498922523054617, -2.229057914452205136, -5.113484796970851676 ) ) ;
#5701=CARTESIAN_POINT ( 'NONE',  ( 46.05330090215556282, 0.2364164235710524975, -5.783357778048662468 ) ) ;
#5703=AXIS2_PLACEMENT_3D ( 'NONE', #3387, #9008, #11529 ) ;
#5705=CARTESIAN_POINT ( 'NONE',  ( 28.97253418081003673, -5.800171738120336151, -7.939653947423662927 ) ) ;
#5720=CARTESIAN_POINT ( 'NONE',  ( 32.96459815279162342, -1.884545423566157174, -4.533357778048659803 ) ) ;
#5722=CARTESIAN_POINT ( 'NONE',  ( 31.58296173575813981, -1.713646710223874381, -6.453230759126465266 ) ) ;
#5725=( BOUNDED_CURVE ( )  B_SPLINE_CURVE ( 2, ( #2039, #15905, #11899, #17482, #3660, #9100, #14641, #15729, #5009 ),
 .UNSPECIFIED., .F., .T. ) 
 B_SPLINE_CURVE_WITH_KNOTS ( ( 3, 2, 2, 2, 3 ),
 ( 0.3653846153846154188, 0.3717948717948718063, 0.3846153846153846367, 0.3974358974358974117, 0.4038461538461538547 ),
 .UNSPECIFIED. ) 
 CURVE ( )  GEOMETRIC_REPRESENTATION_ITEM ( )  RATIONAL_B_SPLINE_CURVE ( ( 0.9330127018922194093, 0.9330127018922196314, 1.000000000000000000, 0.8660254037844387076, 1.000000000000000000, 0.8660254037844387076, 1.000000000000000000, 0.9330127018922190762, 0.9330127018922194093 ) ) 
 REPRESENTATION_ITEM ( '' )  );
#5730=DIRECTION ( 'NONE',  ( -0.1196152422706624058, 0.9928203230275510771, 0.000000000000000000 ) ) ;
#5738=DIRECTION ( 'NONE',  ( 0.9928203230275512992, 0.1196152422706610180, 4.006172263299093133E-17 ) ) ;
#5760=CARTESIAN_POINT ( 'NONE',  ( 38.37070961486131182, 1.238267339652773913, -5.783357778048661579 ) ) ;
#5766=CARTESIAN_POINT ( 'NONE',  ( 30.25524682244395436, -4.391689130744175884, -3.283357778048664688 ) ) ;
#5770=CARTESIAN_POINT ( 'NONE',  ( 31.41114436565740320, -6.133337902414513820, -4.705209693361168455 ) ) ;
#5775=ORIENTED_EDGE ( 'NONE', *, *, #11616, .T. ) ;
#5785=CARTESIAN_POINT ( 'NONE',  ( 29.42285898892238549, -7.010054420087358018, -5.113484796970856117 ) ) ;
#5786=CARTESIAN_POINT ( 'NONE',  ( 29.38830135902312080, -2.615227339812091767, -6.861505862736159145 ) ) ;
#5787=CARTESIAN_POINT ( 'NONE',  ( 29.19631194059803292, -2.001190877926593004, -5.113484796970855228 ) ) ;
#5789=CARTESIAN_POINT ( 'NONE',  ( 26.31556265977298992, -7.384422263489805793, -5.783357778048663356 ) ) ;
#5796=CARTESIAN_POINT ( 'NONE',  ( 31.24973580796908834, -6.452593224933654170, -4.533357778048668685 ) ) ;
#5797=LINE ( 'NONE', #4093, #4543 ) ;
#5800=CARTESIAN_POINT ( 'NONE',  ( 27.08121146544255353, -6.028038774645947839, -7.939653947423662927 ) ) ;
#5808=AXIS2_PLACEMENT_3D ( 'NONE', #1828, #12959, #542 ) ;
#5815=CARTESIAN_POINT ( 'NONE',  ( 31.17093069310692499, -6.462087684996337345, -4.533357778048668685 ) ) ;
#5816=CARTESIAN_POINT ( 'NONE',  ( 31.90644508241650357, -6.373472726347483963, -7.033357778048666908 ) ) ;
#5837=EDGE_CURVE ( 'NONE', #2657, #9429, #16467, .T. ) ;
#5838=( BOUNDED_CURVE ( )  B_SPLINE_CURVE ( 2, ( #2223, #17573, #6376, #844, #10444, #6478, #17382, #3478, #7738 ),
 .UNSPECIFIED., .F., .T. ) 
 B_SPLINE_CURVE_WITH_KNOTS ( ( 3, 2, 2, 2, 3 ),
 ( 0.7884615384615384359, 0.7948717948717948234, 0.8076923076923077094, 0.8205128205128204844, 0.8269230769230769829 ),
 .UNSPECIFIED. ) 
 CURVE ( )  GEOMETRIC_REPRESENTATION_ITEM ( )  RATIONAL_B_SPLINE_CURVE ( ( 0.9330127018922194093, 0.9330127018922194093, 1.000000000000000000, 0.8660254037844387076, 1.000000000000000000, 0.8660254037844387076, 1.000000000000000000, 0.9330127018922187432, 0.9330127018922192983 ) ) 
 REPRESENTATION_ITEM ( '' )  );
#5845=CIRCLE ( 'NONE', #3553, 2.705189185291143605 ) ;
#5850=FACE_OUTER_BOUND ( 'NONE', #6893, .T. ) ;
#5860=CARTESIAN_POINT ( 'NONE',  ( 27.23057351405260818, -1.848475362037681480, -5.783357778048658027 ) ) ;
#5864=CARTESIAN_POINT ( 'NONE',  ( 29.82181869931131146, -4.443908660051686610, -3.627061608673664672 ) ) ;
#5865=( BOUNDED_SURFACE ( )  B_SPLINE_SURFACE ( 1, 2, ( 
 ( #16235, #10581, #5231, #16063, #6437, #2369, #6601, #16330, #8052, #14863, #2451, #2191, #9407, #3808, #2276, #14612, #13231, #14948, #7794, #11958, #808, #6340, #10753, #11864, #2525, #13591, #9326, #17442, #7973, #13421, #1078, #1173, #12225, #5060, #16148, #3709, #9232, #14782, #1000, #4329, #17881, #6957, #4062, #6785, #13765, #16489, #8314, #255, #8406, #2879, #14035, #5674, #9572, #11185, #9842, #16758, #15392, #11280, #6865, #15297, #5766, #5406, #2711, #12396, #12314, #8232, #1343, #13846, #17963, #15124, #5495, #10923, #11017, #2979, #12489, #74, #4163, #16578, #8502, #4244, #7153, #1434, #16858, #2618, #9659, #15209, #16671, #5586, #2791, #1624, #7065, #11103, #9744, #13938, #8147, #1532, #12663, #9491, #15031, #12583, #13678, #162, #1266, #4684, #8585, #7338, #6227, #14121, #17036, #7423, #352, #5860, #17135, #1710, #2075, #10212, #4508, #7599, #7241, #3419, #1981, #15761, #11748, #17231, #4594, #11383, #4771, #14314, #12757, #8687, #10022, #522, #13125, #12938, #10115, #11664, #13027, #15664, #1896, #3335, #8951, #16950, #445, #15570, #10295, #3150, #6037, #3244, #11567, #15845, #14214, #14398, #7505 ),
 ( #14492, #8865, #15485, #1808, #616, #12856, #5947, #704, #8781, #6137, #11471, #4422, #9934, #3066, #6316, #2252, #7770, #2171, #10562, #3511, #7864, #16127, #880, #3689, #13212, #9211, #976, #4949, #6502, #13395, #17417, #11930, #9042, #14672, #3611, #789, #14595, #15940, #12018, #14760, #9133, #7685, #17602, #2345, #16042, #10477, #11839, #13299, #6413, #17518, #5121, #5040, #17317, #4856, #10387, #12601, #6804, #8332, #8520, #1550, #15317, #9762, #11119, #2896, #8167, #273, #1362, #2999, #8425, #12510, #15230, #5603, #1641, #13866, #15146, #13961, #5786, #12415, #15052, #7083, #11205, #17896, #180, #16778, #15413, #10944, #5691, #2730, #4347, #9858, #1282, #14052, #9591, #7173, #12682, #2, #16427, #3992, #6887, #4263, #12331, #2808, #16601, #8251, #5427, #13699, #9508, #2639, #9679, #16508, #4079, #13784, #11036, #5517, #4180, #1452, #6981, #16688, #95, #693, #10010, #11652, #430, #5936, #17219, #1794, #2159, #4758, #4580, #7676, #8673, #3499, #2064, #11461, #10284, #7587, #9031, #15833, #17027, #13113, #14386, #511, #6217, #10103, #8770, #10202, #14480, #11735, #15928, #3406, #8938, #15556, #17308 ) ),
 .UNSPECIFIED., .F., .F., .T. ) 
 B_SPLINE_SURFACE_WITH_KNOTS ( ( 2, 2 ),
 ( 3, 2, 2, 2, 2, 2, 2, 2, 2, 2, 2, 2, 2, 2, 2, 2, 2, 2, 2, 2, 2, 2, 2, 2, 2, 2, 2, 2, 2, 2, 2, 2, 2, 2, 2, 2, 2, 2, 2, 2, 2, 2, 2, 2, 2, 2, 2, 2, 2, 2, 2, 2, 2, 2, 2, 2, 2, 2, 2, 2, 2, 2, 2, 2, 2, 2, 2, 2, 2, 2, 2, 2, 2, 2, 2, 2, 3 ),
 ( 0.000000000000000000, 1.000000000000000000 ),
 ( 0.000000000000000000, 0.01282051282051282007, 0.02564102564102564014, 0.03846153846153846367, 0.05128205128205128027, 0.06410256410256409687, 0.07692307692307692735, 0.08974358974358974395, 0.1025641025641025605, 0.1153846153846153910, 0.1282051282051281937, 0.1410256410256410242, 0.1538461538461538547, 0.1666666666666666574, 0.1794871794871794879, 0.1923076923076923184, 0.2051282051282051211, 0.2179487179487179516, 0.2307692307692307820, 0.2435897435897435848, 0.2564102564102563875, 0.2692307692307692180, 0.2820512820512820484, 0.2948717948717948789, 0.3076923076923077094, 0.3205128205128205399, 0.3333333333333333148, 0.3461538461538461453, 0.3589743589743589758, 0.3717948717948718063, 0.3846153846153846367, 0.3974358974358974117, 0.4102564102564102422, 0.4230769230769230727, 0.4358974358974359031, 0.4487179487179487336, 0.4615384615384615641, 0.4743589743589743390, 0.4871794871794871695, 0.5000000000000000000, 0.5128205128205127750, 0.5256410256410256610, 0.5384615384615384359, 0.5512820512820513219, 0.5641025641025640969, 0.5769230769230768718, 0.5897435897435897578, 0.6025641025641025328, 0.6153846153846154188, 0.6282051282051281937, 0.6410256410256410797, 0.6538461538461538547, 0.6666666666666666297, 0.6794871794871795156, 0.6923076923076922906, 0.7051282051282051766, 0.7179487179487179516, 0.7307692307692307265, 0.7435897435897436125, 0.7564102564102563875, 0.7692307692307692735, 0.7820512820512820484, 0.7948717948717948234, 0.8076923076923077094, 0.8205128205128204844, 0.8333333333333333703, 0.8461538461538461453, 0.8589743589743589203, 0.8717948717948718063, 0.8846153846153845812, 0.8974358974358974672, 0.9102564102564102422, 0.9230769230769231282, 0.9358974358974359031, 0.9487179487179486781, 0.9615384615384615641, 0.9690837704703162414 ),
 .UNSPECIFIED. ) 
 GEOMETRIC_REPRESENTATION_ITEM ( )  RATIONAL_B_SPLINE_SURFACE ( (
 ( 1.000000000000000000, 0.8660254037844387076, 1.000000000000000000, 0.8660254037844387076, 1.000000000000000000, 0.8660254037844387076, 1.000000000000000000, 0.8660254037844387076, 1.000000000000000000, 0.8660254037844387076, 1.000000000000000000, 0.8660254037844387076, 1.000000000000000000, 0.8660254037844387076, 1.000000000000000000, 0.8660254037844387076, 1.000000000000000000, 0.8660254037844387076, 1.000000000000000000, 0.8660254037844387076, 1.000000000000000000, 0.8660254037844387076, 1.000000000000000000, 0.8660254037844387076, 1.000000000000000000, 0.8660254037844387076, 1.000000000000000000, 0.8660254037844387076, 1.000000000000000000, 0.8660254037844387076, 1.000000000000000000, 0.8660254037844387076, 1.000000000000000000, 0.8660254037844387076, 1.000000000000000000, 0.8660254037844387076, 1.000000000000000000, 0.8660254037844387076, 1.000000000000000000, 0.8660254037844387076, 1.000000000000000000, 0.8660254037844387076, 1.000000000000000000, 0.8660254037844387076, 1.000000000000000000, 0.8660254037844387076, 1.000000000000000000, 0.8660254037844387076, 1.000000000000000000, 0.8660254037844387076, 1.000000000000000000, 0.8660254037844387076, 1.000000000000000000, 0.8660254037844387076, 1.000000000000000000, 0.8660254037844387076, 1.000000000000000000, 0.8660254037844387076, 1.000000000000000000, 0.8660254037844387076, 1.000000000000000000, 0.8660254037844387076, 1.000000000000000000, 0.8660254037844387076, 1.000000000000000000, 0.8660254037844387076, 1.000000000000000000, 0.8660254037844387076, 1.000000000000000000, 0.8660254037844387076, 1.000000000000000000, 0.8660254037844387076, 1.000000000000000000, 0.8660254037844387076, 1.000000000000000000, 0.8660254037844387076, 1.000000000000000000, 0.8660254037844387076, 1.000000000000000000, 0.8660254037844387076, 1.000000000000000000, 0.8660254037844387076, 1.000000000000000000, 0.8660254037844387076, 1.000000000000000000, 0.8660254037844387076, 1.000000000000000000, 0.8660254037844387076, 1.000000000000000000, 0.8660254037844387076, 1.000000000000000000, 0.8660254037844387076, 1.000000000000000000, 0.8660254037844387076, 1.000000000000000000, 0.8660254037844387076, 1.000000000000000000, 0.8660254037844387076, 1.000000000000000000, 0.8660254037844387076, 1.000000000000000000, 0.8660254037844387076, 1.000000000000000000, 0.8660254037844387076, 1.000000000000000000, 0.8660254037844387076, 1.000000000000000000, 0.8660254037844387076, 1.000000000000000000, 0.8660254037844387076, 1.000000000000000000, 0.8660254037844387076, 1.000000000000000000, 0.8660254037844387076, 1.000000000000000000, 0.8660254037844387076, 1.000000000000000000, 0.8660254037844387076, 1.000000000000000000, 0.8660254037844387076, 1.000000000000000000, 0.8660254037844387076, 1.000000000000000000, 0.8660254037844387076, 1.000000000000000000, 0.8660254037844387076, 1.000000000000000000, 0.8660254037844387076, 1.000000000000000000, 0.8660254037844387076, 1.000000000000000000, 0.8660254037844387076, 1.000000000000000000, 0.8660254037844387076, 1.000000000000000000, 0.8660254037844387076, 1.000000000000000000, 0.8660254037844387076, 1.000000000000000000, 0.8660254037844387076, 1.000000000000000000, 0.8660254037844387076, 1.000000000000000000, 0.8660254037844387076, 1.000000000000000000, 0.8660254037844387076, 1.000000000000000000, 0.8660254037844387076, 1.000000000000000000, 0.8660254037844387076, 1.000000000000000000, 0.9211513820375816231, 0.9351129643698559146),
 ( 1.000000000000000000, 0.8660254037844387076, 1.000000000000000000, 0.8660254037844387076, 1.000000000000000000, 0.8660254037844387076, 1.000000000000000000, 0.8660254037844387076, 1.000000000000000000, 0.8660254037844387076, 1.000000000000000000, 0.8660254037844387076, 1.000000000000000000, 0.8660254037844387076, 1.000000000000000000, 0.8660254037844387076, 1.000000000000000000, 0.8660254037844387076, 1.000000000000000000, 0.8660254037844387076, 1.000000000000000000, 0.8660254037844387076, 1.000000000000000000, 0.8660254037844387076, 1.000000000000000000, 0.8660254037844387076, 1.000000000000000000, 0.8660254037844387076, 1.000000000000000000, 0.8660254037844387076, 1.000000000000000000, 0.8660254037844387076, 1.000000000000000000, 0.8660254037844387076, 1.000000000000000000, 0.8660254037844387076, 1.000000000000000000, 0.8660254037844387076, 1.000000000000000000, 0.8660254037844387076, 1.000000000000000000, 0.8660254037844387076, 1.000000000000000000, 0.8660254037844387076, 1.000000000000000000, 0.8660254037844387076, 1.000000000000000000, 0.8660254037844387076, 1.000000000000000000, 0.8660254037844387076, 1.000000000000000000, 0.8660254037844387076, 1.000000000000000000, 0.8660254037844387076, 1.000000000000000000, 0.8660254037844387076, 1.000000000000000000, 0.8660254037844387076, 1.000000000000000000, 0.8660254037844387076, 1.000000000000000000, 0.8660254037844387076, 1.000000000000000000, 0.8660254037844387076, 1.000000000000000000, 0.8660254037844387076, 1.000000000000000000, 0.8660254037844387076, 1.000000000000000000, 0.8660254037844387076, 1.000000000000000000, 0.8660254037844387076, 1.000000000000000000, 0.8660254037844387076, 1.000000000000000000, 0.8660254037844387076, 1.000000000000000000, 0.8660254037844387076, 1.000000000000000000, 0.8660254037844387076, 1.000000000000000000, 0.8660254037844387076, 1.000000000000000000, 0.8660254037844387076, 1.000000000000000000, 0.8660254037844387076, 1.000000000000000000, 0.8660254037844387076, 1.000000000000000000, 0.8660254037844387076, 1.000000000000000000, 0.8660254037844387076, 1.000000000000000000, 0.8660254037844387076, 1.000000000000000000, 0.8660254037844387076, 1.000000000000000000, 0.8660254037844387076, 1.000000000000000000, 0.8660254037844387076, 1.000000000000000000, 0.8660254037844387076, 1.000000000000000000, 0.8660254037844387076, 1.000000000000000000, 0.8660254037844387076, 1.000000000000000000, 0.8660254037844387076, 1.000000000000000000, 0.8660254037844387076, 1.000000000000000000, 0.8660254037844387076, 1.000000000000000000, 0.8660254037844387076, 1.000000000000000000, 0.8660254037844387076, 1.000000000000000000, 0.8660254037844387076, 1.000000000000000000, 0.8660254037844387076, 1.000000000000000000, 0.8660254037844387076, 1.000000000000000000, 0.8660254037844387076, 1.000000000000000000, 0.8660254037844387076, 1.000000000000000000, 0.8660254037844387076, 1.000000000000000000, 0.8660254037844387076, 1.000000000000000000, 0.8660254037844387076, 1.000000000000000000, 0.8660254037844387076, 1.000000000000000000, 0.8660254037844387076, 1.000000000000000000, 0.8660254037844387076, 1.000000000000000000, 0.8660254037844387076, 1.000000000000000000, 0.8660254037844387076, 1.000000000000000000, 0.8660254037844387076, 1.000000000000000000, 0.8660254037844387076, 1.000000000000000000, 0.8660254037844387076, 1.000000000000000000, 0.8660254037844387076, 1.000000000000000000, 0.9211513820375816231, 0.9351129643698559146) ) ) 
 REPRESENTATION_ITEM ( '' )  SURFACE ( )  );
#5867=CARTESIAN_POINT ( 'NONE',  ( 26.79905070906539777, -3.354278923027479209, -3.283357778048662023 ) ) ;
#5871=ORIENTED_EDGE ( 'NONE', *, *, #1296, .T. ) ;
#5877=EDGE_CURVE ( 'NONE', #9127, #7301, #3146, .T. ) ;
#5879=CARTESIAN_POINT ( 'NONE',  ( 25.81100034576892455, -6.186289477007987259, -7.540293452860097112 ) ) ;
#5894=CARTESIAN_POINT ( 'NONE',  ( 26.36761712467744090, -6.740983333149474177, -4.705209693361168455 ) ) ;
#5896=ORIENTED_EDGE ( 'NONE', *, *, #16346, .T. ) ;
#5903=VERTEX_POINT ( 'NONE', #16734 ) ;
#5905=ORIENTED_EDGE ( 'NONE', *, *, #15558, .F. ) ;
#5909=CARTESIAN_POINT ( 'NONE',  ( 30.37154917142620292, -2.923863409590206519, -8.283357778048658915 ) ) ;
#5911=ADVANCED_FACE ( 'NONE', ( #16927 ), #5651, .T. ) ;
#5921=CARTESIAN_POINT ( 'NONE',  ( 25.93714794488954212, -2.393855775999666591, -5.783357778048658027 ) ) ;
#5930=CARTESIAN_POINT ( 'NONE',  ( 33.76207435632690590, -3.969185667289998332, -3.627061608673664672 ) ) ;
#5936=CARTESIAN_POINT ( 'NONE',  ( 26.84461768998868436, -2.294720455324902542, -5.783357778048658027 ) ) ;
#5939=CARTESIAN_POINT ( 'NONE',  ( 31.71807556108801407, -1.697368162559112825, -5.113484796970855228 ) ) ;
#5945=DIRECTION ( 'NONE',  ( -0.9928203230275510771, -0.1196152422706614760, -0.000000000000000000 ) ) ;
#5947=CARTESIAN_POINT ( 'NONE',  ( 33.28924367748503244, -4.026152426421394814, -7.939653947423662039 ) ) ;
#5950=CARTESIAN_POINT ( 'NONE',  ( 32.16857880351144416, -6.669052543620333395, -5.783357778048668685 ) ) ;
#5963=CARTESIAN_POINT ( 'NONE',  ( 33.54323074294813267, -5.249493066516778050, -7.939653947423664704 ) ) ;
#5966=CARTESIAN_POINT ( 'NONE',  ( 27.19802975513453092, -2.241944418315925613, -5.783357778048658027 ) ) ;
#5967=CARTESIAN_POINT ( 'NONE',  ( 38.62156597043018991, -0.8438693783906362489, -3.150911402496571867 ) ) ;
#5971=EDGE_LOOP ( 'NONE', ( #5905, #4759, #4781, #8990 ) ) ;
#5978=CARTESIAN_POINT ( 'NONE',  ( 26.98483462626008134, -4.785709214840094816, -7.939653947423662039 ) ) ;
#5979=ORIENTED_EDGE ( 'NONE', *, *, #7750, .T. ) ;
#5993=CARTESIAN_POINT ( 'NONE',  ( 29.14074637024071990, -5.979778010479330774, -3.283357778048667797 ) ) ;
#5996=CARTESIAN_POINT ( 'NONE',  ( 32.50309786422735669, -5.574681056656012323, -8.283357778048662468 ) ) ;
#6004=LINE ( 'NONE', #10182, #14579 ) ;
#6016=PLANE ( 'NONE',  #16204 ) ;
#6017=CARTESIAN_POINT ( 'NONE',  ( 32.72003615946069743, -2.840789625746940938, -7.939653947423660263 ) ) ;
#6027=CARTESIAN_POINT ( 'NONE',  ( 32.51061761821408425, -6.300681867249914525, -4.533357778048668685 ) ) ;
#6033=DIRECTION ( 'NONE',  ( 0.05980762113533059920, -0.4964101615137756496, -0.8660254037844385966 ) ) ;
#6037=CARTESIAN_POINT ( 'NONE',  ( 25.47811240618384687, -2.786519109605914757, -4.533357778048659803 ) ) ;
#6039=CARTESIAN_POINT ( 'NONE',  ( 33.04340326765378677, -1.875050963503474222, -4.533357778048659803 ) ) ;
#6042=CARTESIAN_POINT ( 'NONE',  ( 26.99805802979993885, -6.665027654307603022, -4.705209693361168455 ) ) ;
#6043=EDGE_CURVE ( 'NONE', #3987, #15092, #13167, .T. ) ;
#6044=CARTESIAN_POINT ( 'NONE',  ( 27.15566825608056689, -6.646038734597135011, -4.705209693361169343 ) ) ;
#6048=ORIENTED_EDGE ( 'NONE', *, *, #17743, .T. ) ;
#6056=CARTESIAN_POINT ( 'NONE',  ( 32.29974222271236073, -2.891426744974864071, -3.627061608673662008 ) ) ;
#6068=CARTESIAN_POINT ( 'NONE',  ( 30.42903939560917337, -1.852671564043892660, -5.783357778048658027 ) ) ;
#6071=AXIS2_PLACEMENT_3D ( 'NONE', #11750, #15942, #13127 ) ;
#6073=DIRECTION ( 'NONE',  ( -0.9928203230275510771, -0.1196152422706614760, -0.000000000000000000 ) ) ;
#6076=ORIENTED_EDGE ( 'NONE', *, *, #8060, .F. ) ;
#6079=ORIENTED_EDGE ( 'NONE', *, *, #13273, .F. ) ;
#6090=CARTESIAN_POINT ( 'NONE',  ( 28.69037342443288452, -3.126411886501869741, -3.283357778048662023 ) ) ;
#6093=CARTESIAN_POINT ( 'NONE',  ( 29.67353201968042598, -1.554147106732884920, -5.783357778048658027 ) ) ;
#6103=ORIENTED_EDGE ( 'NONE', *, *, #4015, .T. ) ;
#6115=CARTESIAN_POINT ( 'NONE',  ( 46.86575133767495061, -2.390451368237048513, -5.783357778048661579 ) ) ;
#6121=EDGE_CURVE ( 'NONE', #15406, #14372, #14753, .T. ) ;
#6124=ORIENTED_EDGE ( 'NONE', *, *, #11306, .F. ) ;
#6137=CARTESIAN_POINT ( 'NONE',  ( 33.42946061375642586, -6.517141185936593750, -5.783357778048668685 ) ) ;
#6142=CARTESIAN_POINT ( 'NONE',  ( 29.19137779418881351, -4.519864338893556877, -3.627061608673664672 ) ) ;
#6144=LINE ( 'NONE', #5129, #2629 ) ;
#6149=VERTEX_POINT ( 'NONE', #2713 ) ;
#6157=CARTESIAN_POINT ( 'NONE',  ( 25.62757597683262034, -3.695291012717980994, -7.939653947423660263 ) ) ;
#6164=CARTESIAN_POINT ( 'NONE',  ( 31.20090818012769773, -4.277755612481361602, -8.283357778048662468 ) ) ;
#6176=ORIENTED_EDGE ( 'NONE', *, *, #16826, .T. ) ;
#6177=CARTESIAN_POINT ( 'NONE',  ( 29.91004888286193619, -6.613999042680076990, -4.533357778048668685 ) ) ;
#6187=CARTESIAN_POINT ( 'NONE',  ( 27.49335874655903567, -6.905162478240574053, -7.033357778048666908 ) ) ;
#6188=DIRECTION ( 'NONE',  ( -0.1196152422706610735, 0.9928203230275511881, 0.000000000000000000 ) ) ;
#6190=EDGE_CURVE ( 'NONE', #15926, #13835, #12857, .T. ) ;
#6199=CARTESIAN_POINT ( 'NONE',  ( 31.66250999073069750, -5.675955295111850596, -3.283357778048667797 ) ) ;
#6204=EDGE_LOOP ( 'NONE', ( #17925, #15517, #16396, #6373 ) ) ;
#6211=CARTESIAN_POINT ( 'NONE',  ( 30.18087924896149588, -5.654590020340094725, -3.627061608673668225 ) ) ;
#6212=LINE ( 'NONE', #16111, #4146 ) ;
#6213=CARTESIAN_POINT ( 'NONE',  ( 38.68147913031997831, -1.341155523753223555, -2.283357778048670461 ) ) ;
#6217=CARTESIAN_POINT ( 'NONE',  ( 26.36761712467744090, -6.740983333149474177, -4.705209693361168455 ) ) ;
#6219=ORIENTED_EDGE ( 'NONE', *, *, #1946, .F. ) ;
#6226=CARTESIAN_POINT ( 'NONE',  ( 26.30941689637695902, -7.333411717640721861, -6.290568369890759293 ) ) ;
#6227=CARTESIAN_POINT ( 'NONE',  ( 28.09753128235661279, -6.832371619143005503, -4.533357778048668685 ) ) ;
#6232=CARTESIAN_POINT ( 'NONE',  ( 26.35439372113758694, -4.861664893681965083, -7.939653947423662039 ) ) ;
#6239=VERTEX_POINT ( 'NONE', #4595 ) ;
#6246=CARTESIAN_POINT ( 'NONE',  ( 27.63266882139180680, -2.199775856772564708, -5.783357778048658027 ) ) ;
#6248=CARTESIAN_POINT ( 'NONE',  ( 27.55969062878875064, -7.234529412811931515, -5.783357778048668685 ) ) ;
#6250=CARTESIAN_POINT ( 'NONE',  ( 31.35480929215617252, -6.439933945126671055, -7.033357778048666908 ) ) ;
#6251=EDGE_CURVE ( 'NONE', #13835, #6811, #7610, .T. ) ;
#6255=ORIENTED_EDGE ( 'NONE', *, *, #1638, .T. ) ;
#6258=CARTESIAN_POINT ( 'NONE',  ( 31.54230778485832332, -2.355712103769039611, -4.705209693361160461 ) ) ;
#6259=ORIENTED_EDGE ( 'NONE', *, *, #6823, .T. ) ;
#6266=CARTESIAN_POINT ( 'NONE',  ( 29.11750682573587312, -2.010685337989277954, -5.113484796970851676 ) ) ;
#6275=CARTESIAN_POINT ( 'NONE',  ( 26.31308423962587995, -7.363851090081254824, -5.799730202602000340 ) ) ;
#6278=CARTESIAN_POINT ( 'NONE',  ( 26.55511561737958814, -2.656761491791831187, -7.033357778048658027 ) ) ;
#6279=CARTESIAN_POINT ( 'NONE',  ( 31.38469755857769528, -2.374701023479507178, -4.705209693361161349 ) ) ;
#6280=EDGE_CURVE ( 'NONE', #16733, #4586, #12456, .T. ) ;
#6281=ORIENTED_EDGE ( 'NONE', *, *, #12115, .F. ) ;
#6282=CARTESIAN_POINT ( 'NONE',  ( 30.71189515440122975, -6.854751018602581958, -5.783357778048663356 ) ) ;
#6285=ORIENTED_EDGE ( 'NONE', *, *, #4199, .F. ) ;
#6287=CARTESIAN_POINT ( 'NONE',  ( 31.43732351782677625, -4.249272233123119413, -3.283357778048664688 ) ) ;
#6299=CARTESIAN_POINT ( 'NONE',  ( 30.39102621733566423, -5.629271460726126719, -7.939653947423664704 ) ) ;
#6301=CARTESIAN_POINT ( 'NONE',  ( 25.76466184735054910, -2.811881907026620553, -6.248149982130924762 ) ) ;
#6316=CARTESIAN_POINT ( 'NONE',  ( 32.64557936882268052, -2.222789665795767089, -4.705209693361161349 ) ) ;
#6319=AXIS2_PLACEMENT_3D ( 'NONE', #5569, #2860, #5658 ) ;
#6321=CARTESIAN_POINT ( 'NONE',  ( 28.10549950023366961, -2.142809097641162897, -5.783357778048658027 ) ) ;
#6334=CARTESIAN_POINT ( 'NONE',  ( 29.18947247604338102, -3.066280307211263434, -8.283357778048660691 ) ) ;
#6336=CARTESIAN_POINT ( 'NONE',  ( 29.13014440709066832, -5.781182818409868140, -7.939653947423664704 ) ) ;
#6340=CARTESIAN_POINT ( 'NONE',  ( 32.64947922571280259, -7.010858578292532783, -5.783357778048669573 ) ) ;
#6344=AXIS2_PLACEMENT_3D ( 'NONE', #16491, #5588, #16673 ) ;
#6346=CARTESIAN_POINT ( 'NONE',  ( 32.18597209352066812, -4.159074864394664672, -7.939653947423662039 ) ) ;
#6352=PRODUCT ( 'Bleed Screw Nipple', 'Bleed Screw Nipple', '', ( #12559 ) ) ;
#6354=ORIENTED_EDGE ( 'NONE', *, *, #12904, .T. ) ;
#6359=CARTESIAN_POINT ( 'NONE',  ( 33.64386668575551198, -3.983427357176565486, -8.283357778048662468 ) ) ;
#6363=VECTOR ( 'NONE', #2593, 1000.000000000000114 ) ;
#6369=CARTESIAN_POINT ( 'NONE',  ( 28.01872616749444944, -6.841866079205687790, -4.533357778048668685 ) ) ;
#6371=CARTESIAN_POINT ( 'NONE',  ( 33.28924367748503244, -4.026152426421394814, -7.939653947423662039 ) ) ;
#6373=ORIENTED_EDGE ( 'NONE', *, *, #10552, .T. ) ;
#6376=CARTESIAN_POINT ( 'NONE',  ( 26.63392073224175505, -2.647267031729148012, -7.033357778048658027 ) ) ;
#6393=CARTESIAN_POINT ( 'NONE',  ( 30.41294626588012306, -6.253601060580800564, -6.861505862736167138 ) ) ;
#6403=CARTESIAN_POINT ( 'NONE',  ( 27.48088551392658729, -7.244023872874614689, -5.783357778048657138 ) ) ;
#6408=CARTESIAN_POINT ( 'NONE',  ( 39.19942832275109623, -5.640193629429882449, -1.783357778048662690 ) ) ;
#6413=CARTESIAN_POINT ( 'NONE',  ( 31.08270050955629671, -4.291997302367946077, -3.627061608673664672 ) ) ;
#6416=CARTESIAN_POINT ( 'NONE',  ( 28.38593337277646711, -7.124786616671554107, -5.783357778048668685 ) ) ;
#6424=VECTOR ( 'NONE', #4084, 1000.000000000000227 ) ;
#6431=CARTESIAN_POINT ( 'NONE',  ( 38.64694918415791136, -1.054552983374777098, -1.783357778048662912 ) ) ;
#6432=CARTESIAN_POINT ( 'NONE',  ( 27.48088551392658729, -7.244023872874614689, -5.783357778048657138 ) ) ;
#6433=CARTESIAN_POINT ( 'NONE',  ( 31.06530721954707985, -6.801974981593605030, -5.783357778048669573 ) ) ;
#6437=CARTESIAN_POINT ( 'NONE',  ( 32.93832978346670615, -1.887710243310447567, -7.033357778048658027 ) ) ;
#6445=CARTESIAN_POINT ( 'NONE',  ( 31.06530721954707985, -6.801974981593605918, -5.783357778048669573 ) ) ;
#6448=CARTESIAN_POINT ( 'NONE',  ( 38.37070961486131182, 1.238267339652773913, -5.783357778048661579 ) ) ;
#6463=AXIS2_PLACEMENT_3D ( 'NONE', #17200, #3120, #15816 ) ;
#6470=ORIENTED_EDGE ( 'NONE', *, *, #11504, .T. ) ;
#6471=CARTESIAN_POINT ( 'NONE',  ( 28.44643833274707845, -2.428894455266221275, -7.033357778048658027 ) ) ;
#6472=CARTESIAN_POINT ( 'NONE',  ( 31.93198502805756789, -2.935734224299280548, -7.939653947423660263 ) ) ;
#6478=CARTESIAN_POINT ( 'NONE',  ( 26.90793483298705979, -6.248787706170159773, -8.283357778048664244 ) ) ;
#6479=VERTEX_POINT ( 'NONE', #9807 ) ;
#6489=CARTESIAN_POINT ( 'NONE',  ( 28.26310972651430120, -2.123820177930694442, -5.783357778048658027 ) ) ;
#6490=CARTESIAN_POINT ( 'NONE',  ( 32.97402322492378346, -4.064130265842336165, -3.627061608673664672 ) ) ;
#6502=CARTESIAN_POINT ( 'NONE',  ( 31.91006497951310550, -2.311404624444611589, -6.861505862736159145 ) ) ;
#6523=CARTESIAN_POINT ( 'NONE',  ( 29.97942892559193950, -4.424919740341219487, -3.627061608673664672 ) ) ;
#6531=CARTESIAN_POINT ( 'NONE',  ( 31.24031073583692475, -4.273008382657478954, -3.627061608673664672 ) ) ;
#6534=CARTESIAN_POINT ( 'NONE',  ( 26.01652455409633902, -4.902371455920936150, -5.783357778048664244 ) ) ;
#6548=CARTESIAN_POINT ( 'NONE',  ( 30.98067518586950442, -1.786210345264705790, -5.783357778048658027 ) ) ;
#6550=CARTESIAN_POINT ( 'NONE',  ( 32.34358231980129261, -4.140085944684206432, -3.627061608673664672 ) ) ;
#6553=LINE ( 'NONE', #10613, #1179 ) ;
#6559=( BOUNDED_CURVE ( )  B_SPLINE_CURVE ( 2, ( #14592, #13122, #14670, #12100, #1057, #6578, #876, #14488, #10560 ),
 .UNSPECIFIED., .F., .T. ) 
 B_SPLINE_CURVE_WITH_KNOTS ( ( 3, 2, 2, 2, 3 ),
 ( 0.6346153846153846922, 0.6410256410256410797, 0.6538461538461538547, 0.6666666666666666297, 0.6730769230769231282 ),
 .UNSPECIFIED. ) 
 CURVE ( )  GEOMETRIC_REPRESENTATION_ITEM ( )  RATIONAL_B_SPLINE_CURVE ( ( 0.9330127018922192983, 0.9330127018922198534, 1.000000000000000000, 0.8660254037844387076, 1.000000000000000000, 0.8660254037844387076, 1.000000000000000000, 0.9330127018922187432, 0.9330127018922192983 ) ) 
 REPRESENTATION_ITEM ( '' )  );
#6564=CARTESIAN_POINT ( 'NONE',  ( 29.17398450417959310, -7.029842018119214941, -5.783357778048669573 ) ) ;
#6565=CARTESIAN_POINT ( 'NONE',  ( 25.95846283556874212, -3.455553161483297053, -8.283357778048660691 ) ) ;
#6569=( BOUNDED_CURVE ( )  B_SPLINE_CURVE ( 2, ( #14689, #11953, #2446, #3528, #17621, #5140, #7969, #13501, #6597 ),
 .UNSPECIFIED., .F., .T. ) 
 B_SPLINE_CURVE_WITH_KNOTS ( ( 3, 2, 2, 2, 3 ),
 ( 0.4038461538461538547, 0.4102564102564102422, 0.4230769230769230727, 0.4358974358974359031, 0.4423076923076923461 ),
 .UNSPECIFIED. ) 
 CURVE ( )  GEOMETRIC_REPRESENTATION_ITEM ( )  RATIONAL_B_SPLINE_CURVE ( ( 0.9330127018922194093, 0.9330127018922196314, 1.000000000000000000, 0.8660254037844387076, 1.000000000000000000, 0.8660254037844387076, 1.000000000000000000, 0.9330127018922190762, 0.9330127018922194093 ) ) 
 REPRESENTATION_ITEM ( '' )  );
#6570=AXIS2_PLACEMENT_3D ( 'NONE', #14822, #3936, #9115 ) ;
#6578=CARTESIAN_POINT ( 'NONE',  ( 28.16881664323204859, -6.096876348486420127, -8.283357778048664244 ) ) ;
#6590=ORIENTED_EDGE ( 'NONE', *, *, #340, .T. ) ;
#6597=CARTESIAN_POINT ( 'NONE',  ( 30.08145424927873535, -6.930706697444451336, -5.783357778048663356 ) ) ;
#6599=CARTESIAN_POINT ( 'NONE',  ( 30.81132015408399027, -5.578634341498224458, -3.627061608673668225 ) ) ;
#6601=CARTESIAN_POINT ( 'NONE',  ( 33.09223089549517738, -4.049888575955752579, -8.283357778048662468 ) ) ;
#6609=CARTESIAN_POINT ( 'NONE',  ( 32.91278983782564183, -5.325448745358647429, -7.939653947423662927 ) ) ;
#6623=CYLINDRICAL_SURFACE ( 'NONE', #16867, 2.500000000000001776 ) ;
#6633=CARTESIAN_POINT ( 'NONE',  ( 26.24565837299761739, -7.163851760794091916, -7.234565377303040279 ) ) ;
#6634=CARTESIAN_POINT ( 'NONE',  ( 31.49429780130001788, -5.496349022752856861, -7.939653947423662927 ) ) ;
#6636=CARTESIAN_POINT ( 'NONE',  ( 32.34167700165585302, -2.686501913001913433, -8.283357778048660691 ) ) ;
#6648=CARTESIAN_POINT ( 'NONE',  ( 26.01595305975170547, -2.384361315936983416, -5.783357778048670461 ) ) ;
#6650=CARTESIAN_POINT ( 'NONE',  ( 28.08810621022444920, -4.652786776866828511, -3.627061608673664672 ) ) ;
#6661=ORIENTED_EDGE ( 'NONE', *, *, #3647, .F. ) ;
#6670=CARTESIAN_POINT ( 'NONE',  ( 28.13873763417255347, -3.192873105281056390, -3.283357778048662023 ) ) ;
#6680=ORIENTED_EDGE ( 'NONE', *, *, #10725, .F. ) ;
#6682=CARTESIAN_POINT ( 'NONE',  ( 28.82057243903374655, -7.082618055128190093, -5.783357778048668685 ) ) ;
#6684=ORIENTED_EDGE ( 'NONE', *, *, #7138, .F. ) ;
#6690=CARTESIAN_POINT ( 'NONE',  ( 26.21851383115118495, -6.578905779530963116, -7.633279253667162756 ) ) ;
#6691=LINE ( 'NONE', #3976, #9639 ) ;
#6692=DIRECTION ( 'NONE',  ( -0.1196152422706610735, 0.9928203230275511881, 0.000000000000000000 ) ) ;
#6698=CARTESIAN_POINT ( 'NONE',  ( 29.55043834383900148, -5.730545699181964991, -3.627061608673668225 ) ) ;
#6702=ORIENTED_EDGE ( 'NONE', *, *, #419, .F. ) ;
#6707=CARTESIAN_POINT ( 'NONE',  ( 32.55256711014040150, -6.632986398338614364, -6.453230759126470595 ) ) ;
#6708=DIRECTION ( 'NONE',  ( -0.05980762113533041185, 0.4964101615137757606, -0.8660254037844384856 ) ) ;
#6721=CARTESIAN_POINT ( 'NONE',  ( 28.35948656569676629, -3.366149737736551906, -3.627061608673662896 ) ) ;
#6741=CARTESIAN_POINT ( 'NONE',  ( 33.79776779778399032, -6.145605689821873163, -7.033357778048666908 ) ) ;
#6742=EDGE_CURVE ( 'NONE', #17907, #2702, #4077, .T. ) ;
#6746=ORIENTED_EDGE ( 'NONE', *, *, #11581, .T. ) ;
#6754=ORIENTED_EDGE ( 'NONE', *, *, #16115, .T. ) ;
#6759=ORIENTED_EDGE ( 'NONE', *, *, #10386, .T. ) ;
#6768=CARTESIAN_POINT ( 'NONE',  ( 25.89690931182567724, -3.909551132893385184, -5.783357778048664244 ) ) ;
#6781=ORIENTED_EDGE ( 'NONE', *, *, #2157, .F. ) ;
#6783=CARTESIAN_POINT ( 'NONE',  ( 26.01595305975170547, -2.384361315936983416, -5.783357778048670461 ) ) ;
#6785=CARTESIAN_POINT ( 'NONE',  ( 31.32102116884452414, -5.717097954277069682, -8.283357778048662468 ) ) ;
#6786=DIRECTION ( 'NONE',  ( -0.1196152422706610735, 0.9928203230275511881, 0.000000000000000000 ) ) ;
#6793=CARTESIAN_POINT ( 'NONE',  ( 27.25621498173240198, -3.499072175709823984, -3.627061608673662008 ) ) ;
#6798=VERTEX_POINT ( 'NONE', #12247 ) ;
#6804=CARTESIAN_POINT ( 'NONE',  ( 30.88577694472199298, -6.196634301449400084, -6.861505862736166250 ) ) ;
#6809=UNCERTAINTY_MEASURE_WITH_UNIT (LENGTH_MEASURE( 1.000000000000000082E-05 ), #9663, 'distance_accuracy_value', 'NONE');
#6811=VERTEX_POINT ( 'NONE', #5601 ) ;
#6818=CARTESIAN_POINT ( 'NONE',  ( 29.51982165028991645, -6.361204938940122844, -4.705209693361168455 ) ) ;
#6820=CARTESIAN_POINT ( 'NONE',  ( 32.46178999037268653, -4.125844254797621957, -8.283357778048662468 ) ) ;
#6823=EDGE_CURVE ( 'NONE', #4105, #6239, #12130, .T. ) ;
#6831=CARTESIAN_POINT ( 'NONE',  ( 27.88665588685489993, -3.423116496867954162, -3.627061608673662008 ) ) ;
#6862=CARTESIAN_POINT ( 'NONE',  ( 26.27749392786456895, -6.324743385012030927, -8.283357778048664244 ) ) ;
#6865=CARTESIAN_POINT ( 'NONE',  ( 30.61929490284659394, -6.528548903775525325, -4.533357778048668685 ) ) ;
#6866=LINE ( 'NONE', #11019, #12810 ) ;
#6867=CIRCLE ( 'NONE', #12066, 2.499999999999999556 ) ;
#6870=SHAPE_REPRESENTATION_RELATIONSHIP ( 'NONE' , 'NONE' ,  #2651, #7664 ) ;
#6872=CARTESIAN_POINT ( 'NONE',  ( 27.45766530510195835, -4.728742455708699666, -3.627061608673664672 ) ) ;
#6879=ORIENTED_EDGE ( 'NONE', *, *, #15699, .F. ) ;
#6885=VERTEX_POINT ( 'NONE', #14330 ) ;
#6887=CARTESIAN_POINT ( 'NONE',  ( 28.23249303296521617, -2.754479417688857179, -4.705209693361161349 ) ) ;
#6889=DIRECTION ( 'NONE',  ( 0.9928203230275510771, 0.1196152422706609902, 4.006172263299092517E-17 ) ) ;
#6893=EDGE_LOOP ( 'NONE', ( #6079, #8981, #18, #4844 ) ) ;
#6897=CARTESIAN_POINT ( 'NONE',  ( 33.66004903264009585, -1.463398710186758267, -5.783357778048663356 ) ) ;
#6899=FACE_OUTER_BOUND ( 'NONE', #6204, .T. ) ;
#6901=CARTESIAN_POINT ( 'NONE',  ( 27.61527553138257574, -4.709753535998224550, -7.939653947423662039 ) ) ;
#6906=AXIS2_PLACEMENT_3D ( 'NONE', #8581, #247, #6951 ) ;
#6915=CARTESIAN_POINT ( 'NONE',  ( 27.23882169172318513, -6.009049854935478052, -7.939653947423664704 ) ) ;
#6931=CARTESIAN_POINT ( 'NONE',  ( 46.86575133767495061, -2.390451368237048069, -5.783357778048661579 ) ) ;
#6940=AXIS2_PLACEMENT_3D ( 'NONE', #4416, #9837, #6033 ) ;
#6951=DIRECTION ( 'NONE',  ( 0.1196152422706608098, -0.9928203230275511881, 0.000000000000000000 ) ) ;
#6954=CARTESIAN_POINT ( 'NONE',  ( 27.12922144900085186, -2.887401855662130146, -4.705209693361160461 ) ) ;
#6955=CARTESIAN_POINT ( 'NONE',  ( 26.02974819644417792, -2.720057890826728109, -4.533357778048659803 ) ) ;
#6957=CARTESIAN_POINT ( 'NONE',  ( 31.08079519141086777, -2.838413270685653078, -8.283357778048658915 ) ) ;
#6963=FILL_AREA_STYLE_COLOUR ( '', #11281 ) ;
#6964=CARTESIAN_POINT ( 'NONE',  ( 30.13703915187255689, -4.405930820630744371, -7.939653947423662039 ) ) ;
#6967=AXIS2_PLACEMENT_3D ( 'NONE', #8203, #16542, #12093 ) ;
#6968=CARTESIAN_POINT ( 'NONE',  ( 29.03376756790819613, -4.538853258604016006, -7.939653947423662039 ) ) ;
#6969=VECTOR ( 'NONE', #16282, 1000.000000000000227 ) ;
#6980=CARTESIAN_POINT ( 'NONE',  ( 28.63031693179632242, -2.406740715396564756, -4.533357778048659803 ) ) ;
#6981=CARTESIAN_POINT ( 'NONE',  ( 27.73357241910951743, -6.576412695658750529, -6.861505862736166250 ) ) ;
#6982=CARTESIAN_POINT ( 'NONE',  ( 29.84999239022537409, -5.894327871574777333, -3.283357778048667797 ) ) ;
#6985=CARTESIAN_POINT ( 'NONE',  ( 28.16197717867739314, -7.161965777771100328, -5.113484796970856117 ) ) ;
#6986=EDGE_CURVE ( 'NONE', #16315, #4277, #6569, .T. ) ;
#6993=DIRECTION ( 'NONE',  ( 0.7866107318554522720, -0.6174492339697490451, 8.659560562354985860E-17 ) ) ;
#6995=CARTESIAN_POINT ( 'NONE',  ( 28.10549950023367316, -2.142809097641162897, -5.783357778048658915 ) ) ;
#7000=CARTESIAN_POINT ( 'NONE',  ( 32.32036211097666012, -1.624804527518282748, -5.783357778048663356 ) ) ;
#7016=CARTESIAN_POINT ( 'NONE',  ( 26.51200394741821498, -4.842675973971495296, -7.939653947423662039 ) ) ;
#7022=EDGE_CURVE ( 'NONE', #15625, #8115, #4717, .T. ) ;
#7033=FILL_AREA_STYLE ('',( #4390 ) ) ;
#7038=EDGE_CURVE ( 'NONE', #15016, #9716, #14776, .T. ) ;
#7050=ORIENTED_EDGE ( 'NONE', *, *, #6280, .T. ) ;
#7059=DIRECTION ( 'NONE',  ( 0.7020299829125996594, 0.08458074894285612377, 0.7071067811865480168 ) ) ;
#7060=CARTESIAN_POINT ( 'NONE',  ( 27.45766530510195835, -4.728742455708699666, -3.627061608673664672 ) ) ;
#7061=AXIS2_PLACEMENT_3D ( 'NONE', #16705, #12525, #10058 ) ;
#7065=CARTESIAN_POINT ( 'NONE',  ( 28.67914455963771303, -4.581578327848842669, -8.283357778048662468 ) ) ;
#7067=CARTESIAN_POINT ( 'NONE',  ( 32.06776442294927421, -4.173316554281249147, -3.283357778048664688 ) ) ;
#7070=CARTESIAN_POINT ( 'NONE',  ( 32.51858583609114106, -1.611119345748072362, -5.783357778048658027 ) ) ;
#7071=EDGE_CURVE ( 'NONE', #2203, #17907, #4876, .T. ) ;
#7072=CARTESIAN_POINT ( 'NONE',  ( 28.91547068018125799, -2.672194098943493135, -6.861505862736158257 ) ) ;
#7075=VERTEX_POINT ( 'NONE', #7788 ) ;
#7082=CARTESIAN_POINT ( 'NONE',  ( 33.78529456515154550, -6.484467084455914687, -5.783357778048663356 ) ) ;
#7083=CARTESIAN_POINT ( 'NONE',  ( 29.60297508593253468, -5.724216059278466773, -7.939653947423664704 ) ) ;
#7096=CARTESIAN_POINT ( 'NONE',  ( 26.86653773853314320, -2.919050055179571945, -6.861505862736159145 ) ) ;
#7106=EDGE_CURVE ( 'NONE', #12046, #3520, #4158, .T. ) ;
#7114=ORIENTED_EDGE ( 'NONE', *, *, #17743, .F. ) ;
#7115=CARTESIAN_POINT ( 'NONE',  ( 31.07327543742414022, -2.112412460091767308, -4.533357778048659803 ) ) ;
#7122=ORIENTED_EDGE ( 'NONE', *, *, #2538, .T. ) ;
#7127=EDGE_LOOP ( 'NONE', ( #5373, #554, #9221 ) ) ;
#7133=( BOUNDED_CURVE ( )  B_SPLINE_CURVE ( 2, ( #7497, #10378, #13020, #7855, #15932, #3503, #9035, #2163, #6403 ),
 .UNSPECIFIED., .F., .T. ) 
 B_SPLINE_CURVE_WITH_KNOTS ( ( 3, 2, 2, 2, 3 ),
 ( 0.7884615384615384359, 0.7948717948717948234, 0.8076923076923077094, 0.8205128205128204844, 0.8269230769230769829 ),
 .UNSPECIFIED. ) 
 CURVE ( )  GEOMETRIC_REPRESENTATION_ITEM ( )  RATIONAL_B_SPLINE_CURVE ( ( 0.9330127018922194093, 0.9330127018922194093, 1.000000000000000000, 0.8660254037844387076, 1.000000000000000000, 0.8660254037844387076, 1.000000000000000000, 0.9330127018922187432, 0.9330127018922192983 ) ) 
 REPRESENTATION_ITEM ( '' )  );
#7134=CARTESIAN_POINT ( 'NONE',  ( 32.93832978346670615, -1.887710243310447567, -7.033357778048658027 ) ) ;
#7138=EDGE_CURVE ( 'NONE', #2767, #7075, #2296, .T. ) ;
#7144=CARTESIAN_POINT ( 'NONE',  ( 34.51156627690993162, -8.531090163810741700, -5.783357778048662468 ) ) ;
#7147=DIRECTION ( 'NONE',  ( 0.9928203230275512992, 0.1196152422706610180, 4.006172263299093133E-17 ) ) ;
#7152=ORIENTED_EDGE ( 'NONE', *, *, #3627, .F. ) ;
#7153=CARTESIAN_POINT ( 'NONE',  ( 29.46348657678868577, -6.667800981652280967, -7.033357778048666908 ) ) ;
#7157=CARTESIAN_POINT ( 'NONE',  ( 31.88814493096863956, -1.687075024589942851, -5.783357778048658027 ) ) ;
#7160=CARTESIAN_POINT ( 'NONE',  ( 27.26074174026764751, -6.633379454790151009, -6.861505862736167138 ) ) ;
#7173=CARTESIAN_POINT ( 'NONE',  ( 29.01637427789896151, -7.048830937829683840, -5.783357778048668685 ) ) ;
#7174=CARTESIAN_POINT ( 'NONE',  ( 29.39961944441754227, -3.040961747597316744, -3.283357778048662023 ) ) ;
#7184=DIRECTION ( 'NONE',  ( 0.9928203230275512992, 0.1196152422706607682, -0.000000000000000000 ) ) ;
#7187=CARTESIAN_POINT ( 'NONE',  ( 26.24062359194589433, -6.129313013101782559, -3.627061608673667781 ) ) ;
#7189=VERTEX_POINT ( 'NONE', #16573 ) ;
#7190=CARTESIAN_POINT ( 'NONE',  ( 26.01652455409633902, -4.902371455920926380, -5.783357778048663356 ) ) ;
#7191=CARTESIAN_POINT ( 'NONE',  ( 46.98536657994561949, -3.383271691264599035, -5.783357778048662468 ) ) ;
#7193=ORIENTED_EDGE ( 'NONE', *, *, #13165, .T. ) ;
#7200=CARTESIAN_POINT ( 'NONE',  ( 30.08145424927873535, -6.930706697444451336, -5.783357778048663356 ) ) ;
#7203=CARTESIAN_POINT ( 'NONE',  ( 30.93441382992541477, -1.402235749049144609, -5.783357778048658027 ) ) ;
#7223=CARTESIAN_POINT ( 'NONE',  ( 32.70264286945147347, -5.350767304972614546, -3.627061608673668225 ) ) ;
#7238=CARTESIAN_POINT ( 'NONE',  ( 39.47566789204768867, -7.933013952457433682, -5.783357778048662468 ) ) ;
#7241=CARTESIAN_POINT ( 'NONE',  ( 27.46709037723411839, -6.908327297984874882, -4.533357778048668685 ) ) ;
#7245=CARTESIAN_POINT ( 'NONE',  ( 30.45225960443380231, -4.367952981209816343, -3.627061608673664672 ) ) ;
#7247=CARTESIAN_POINT ( 'NONE',  ( 25.96814307759224150, -4.500799614243312874, -8.119953194407841579 ) ) ;
#7250=ORIENTED_EDGE ( 'NONE', *, *, #2538, .F. ) ;
#7258=CARTESIAN_POINT ( 'NONE',  ( 33.32855701603872234, -2.140504347050403045, -6.861505862736158257 ) ) ;
#7261=FACE_OUTER_BOUND ( 'NONE', #11043, .T. ) ;
#7264=CARTESIAN_POINT ( 'NONE',  ( 28.11132641904908169, -7.168068194032743534, -5.783357778048668685 ) ) ;
#7284=DIRECTION ( 'NONE',  ( 0.1196152422706618645, -0.9928203230275510771, 0.000000000000000000 ) ) ;
#7289=DIRECTION ( 'NONE',  ( 0.1196152422706609625, -0.9928203230275510771, -0.000000000000000000 ) ) ;
#7291=CARTESIAN_POINT ( 'NONE',  ( 30.80688261270428541, -4.325227911964988792, -3.283357778048664688 ) ) ;
#7292=CARTESIAN_POINT ( 'NONE',  ( 31.87265695910486230, -5.650636735497883478, -8.283357778048664244 ) ) ;
#7297=CARTESIAN_POINT ( 'NONE',  ( 30.40088504037531791, -1.856063607844930852, -6.453230759126464378 ) ) ;
#7301=VERTEX_POINT ( 'NONE', #1803 ) ;
#7320=ADVANCED_FACE ( 'NONE', ( #12751 ), #12850, .F. ) ;
#7330=ORIENTED_EDGE ( 'NONE', *, *, #7138, .T. ) ;
#7334=ORIENTED_EDGE ( 'NONE', *, *, #16942, .F. ) ;
#7336=DIRECTION ( 'NONE',  ( 0.9928203230275511881, 0.1196152422706610735, 9.614813431917827710E-17 ) ) ;
#7338=CARTESIAN_POINT ( 'NONE',  ( 28.23639288985533824, -7.542548330185622874, -5.783357778048669573 ) ) ;
#7339=CARTESIAN_POINT ( 'NONE',  ( 33.68326924318660076, -3.978680127145231893, -3.283357778048664688 ) ) ;
#7342=CARTESIAN_POINT ( 'NONE',  ( 29.99682221560115991, -1.914942061115552541, -5.783357778048658027 ) ) ;
#7358=CARTESIAN_POINT ( 'NONE',  ( 25.83772294520678159, -3.669972453104032084, -3.627061608673662896 ) ) ;
#7369=DIRECTION ( 'NONE',  ( -0.1196152422706599633, 0.9928203230275514102, 0.000000000000000000 ) ) ;
#7371=CARTESIAN_POINT ( 'NONE',  ( 26.88845778707760914, -3.543379655034240905, -7.939653947423660263 ) ) ;
#7373=ADVANCED_FACE ( 'NONE', ( #612 ), #1893, .T. ) ;
#7374=ADVANCED_FACE ( 'NONE', ( #9930 ), #10209, .T. ) ;
#7382=B_SPLINE_CURVE_WITH_KNOTS ( 'NONE', 3,
 ( #12943, #450, #14405, #10029, #13035, #16764, #8508, #7247, #11390, #9847, #12763, #10121, #7512, #15491, #15766, #4691, #1986, #16865 ),
 .UNSPECIFIED., .F., .F.,
 ( 4, 2, 2, 2, 2, 2, 2, 2, 4 ),
 ( 0.000000000000000000, 0.0005705796246920901435, 0.001141159249384180287, 0.001711738874076270539, 0.002282318498768360574, 0.002852898123460450609, 0.003423477748152541078, 0.003994057372844630679, 0.004564636997536721148 ),
 .UNSPECIFIED. ) ;
#7388=CARTESIAN_POINT ( 'NONE',  ( 31.12210306526553083, -4.287250072544045665, -8.283357778048662468 ) ) ;
#7401=VERTEX_POINT ( 'NONE', #2166 ) ;
#7403=CARTESIAN_POINT ( 'NONE',  ( 34.51156627690993162, -8.531090163810741700, -5.783357778048662468 ) ) ;
#7408=CARTESIAN_POINT ( 'NONE',  ( 32.91278983782564183, -5.325448745358647429, -7.939653947423664704 ) ) ;
#7423=CARTESIAN_POINT ( 'NONE',  ( 27.50829672905005907, -3.268828784122927100, -3.283357778048662023 ) ) ;
#7426=CARTESIAN_POINT ( 'NONE',  ( 26.98483462626008134, -4.785709214840094816, -7.939653947423662039 ) ) ;
#7434=FACE_OUTER_BOUND ( 'NONE', #17162, .T. ) ;
#7437=CARTESIAN_POINT ( 'NONE',  ( 32.30426898124760982, -6.025734024055190652, -6.861505862736167138 ) ) ;
#7439=CARTESIAN_POINT ( 'NONE',  ( 27.41826274939272423, -4.733489685532582314, -8.283357778048662468 ) ) ;
#7441=CARTESIAN_POINT ( 'NONE',  ( 27.73348320195396965, -4.695511846111656062, -3.283357778048664688 ) ) ;
#7465=CARTESIAN_POINT ( 'NONE',  ( 27.21934464581372737, -3.303641803799556964, -8.283357778048658915 ) ) ;
#7469=AXIS2_PLACEMENT_3D ( 'NONE', #12632, #220, #5730 ) ;
#7474=ORIENTED_EDGE ( 'NONE', *, *, #9395, .T. ) ;
#7475=CARTESIAN_POINT ( 'NONE',  ( 28.11132641904908169, -7.168068194032743534, -5.783357778048668685 ) ) ;
#7478=CARTESIAN_POINT ( 'NONE',  ( 26.61898274975073164, -6.283600725846810953, -3.283357778048667797 ) ) ;
#7479=CARTESIAN_POINT ( 'NONE',  ( 30.63309003953906995, -6.864245478665264244, -5.783357778048663356 ) ) ;
#7485=CARTESIAN_POINT ( 'NONE',  ( 32.50119254608192421, -4.121097024973739309, -3.627061608673664672 ) ) ;
#7497=CARTESIAN_POINT ( 'NONE',  ( 27.19802975513453092, -2.241944418315925613, -5.783357778048658027 ) ) ;
#7505=CARTESIAN_POINT ( 'NONE',  ( 25.63782166807609997, -6.407846580969937200, -7.820349034508990549 ) ) ;
#7508=CARTESIAN_POINT ( 'NONE',  ( 26.46816385032927599, -3.594016774262162706, -3.627061608673662896 ) ) ;
#7509=ORIENTED_EDGE ( 'NONE', *, *, #10513, .F. ) ;
#7512=CARTESIAN_POINT ( 'NONE',  ( 25.83183225892938140, -3.369404079293177645, -7.443282702368841264 ) ) ;
#7515=EDGE_LOOP ( 'NONE', ( #1594, #135, #2047, #3582 ) ) ;
#7519=ORIENTED_EDGE ( 'NONE', *, *, #13177, .T. ) ;
#7526=CARTESIAN_POINT ( 'NONE',  ( 26.24062359194589078, -6.129313013101781671, -3.627061608673667781 ) ) ;
#7528=DIRECTION ( 'NONE',  ( -0.9928203230275512992, -0.1196152422706610180, -9.614813431917824012E-17 ) ) ;
#7531=CARTESIAN_POINT ( 'NONE',  ( 38.94468999590795733, -1.453587954722214137, -2.531230242176644829 ) ) ;
#7532=CARTESIAN_POINT ( 'NONE',  ( 28.13948077428293715, -7.164676150231702678, -6.453230759126474148 ) ) ;
#7535=ADVANCED_FACE ( 'NONE', ( #874 ), #17514, .F. ) ;
#7548=VECTOR ( 'NONE', #5551, 1000.000000000000114 ) ;
#7551=CARTESIAN_POINT ( 'NONE',  ( 29.86122125502053848, -4.439161430227785310, -8.283357778048662468 ) ) ;
#7557=CARTESIAN_POINT ( 'NONE',  ( 28.69037342443288452, -3.126411886501869741, -3.283357778048662023 ) ) ;
#7565=CARTESIAN_POINT ( 'NONE',  ( 30.57046727500519978, -4.353711291323232757, -8.283357778048662468 ) ) ;
#7570=CARTESIAN_POINT ( 'NONE',  ( 25.87953856062030766, -3.765371892057810754, -3.950981403410641857 ) ) ;
#7574=ADVANCED_FACE ( 'NONE', ( #4032 ), #12158, .T. ) ;
#7579=CARTESIAN_POINT ( 'NONE',  ( 31.55553118839817728, -4.235030543236534939, -7.939653947423662039 ) ) ;
#7587=CARTESIAN_POINT ( 'NONE',  ( 26.21417678486618641, -2.370676134166772808, -5.783357778048658027 ) ) ;
#7593=ORIENTED_EDGE ( 'NONE', *, *, #12167, .T. ) ;
#7595=AXIS2_PLACEMENT_3D ( 'NONE', #14161, #478, #7284 ) ;
#7597=LINE ( 'NONE', #972, #17755 ) ;
#7599=CARTESIAN_POINT ( 'NONE',  ( 27.60595198473284384, -7.618504009027492252, -5.783357778048669573 ) ) ;
#7601=AXIS2_PLACEMENT_3D ( 'NONE', #8678, #4676, #15561 ) ;
#7603=CARTESIAN_POINT ( 'NONE',  ( 26.25801688195511474, -3.619335333876111171, -7.939653947423660263 ) ) ;
#7610=( BOUNDED_CURVE ( )  B_SPLINE_CURVE ( 2, ( #3151, #16859, #6039, #1711, #16952 ),
 .UNSPECIFIED., .F., .T. ) 
 B_SPLINE_CURVE_WITH_KNOTS ( ( 3, 2, 3 ),
 ( 0.000000000000000000, 0.01282051282051282007, 0.01923076923076924571 ),
 .UNSPECIFIED. ) 
 CURVE ( )  GEOMETRIC_REPRESENTATION_ITEM ( )  RATIONAL_B_SPLINE_CURVE ( ( 1.000000000000000000, 0.8660254037844387076, 1.000000000000000000, 0.9330127018922191873, 0.9330127018922194093 ) ) 
 REPRESENTATION_ITEM ( '' )  );
#7613=AXIS2_PLACEMENT_3D ( 'NONE', #11373, #14026, #11558 ) ;
#7619=CARTESIAN_POINT ( 'NONE',  ( 32.93018312783485158, -2.815471066132994249, -3.627061608673662008 ) ) ;
#7620=CARTESIAN_POINT ( 'NONE',  ( 30.64556327217151122, -6.525384084031224496, -7.033357778048666908 ) ) ;
#7630=VECTOR ( 'NONE', #16949, 1000.000000000000227 ) ;
#7631=CARTESIAN_POINT ( 'NONE',  ( 32.81641299864316608, -4.083119185552795294, -7.939653947423662039 ) ) ;
#7640=EDGE_CURVE ( 'NONE', #7189, #317, #16464, .T. ) ;
#7651=DIRECTION ( 'NONE',  ( -0.1196152422706584506, 0.9928203230275515212, 0.000000000000000000 ) ) ;
#7652=CARTESIAN_POINT ( 'NONE',  ( 29.70732014299206369, -2.276983097582480742, -7.033357778048658027 ) ) ;
#7654=VERTEX_POINT ( 'NONE', #2588 ) ;
#7659=PLANE ( 'NONE',  #6463 ) ;
#7660=CARTESIAN_POINT ( 'NONE',  ( 31.07327543742414022, -2.112412460091767308, -4.533357778048659803 ) ) ;
#7664=ADVANCED_BREP_SHAPE_REPRESENTATION ( '', ( #17610, #3575 ), #12173 ) ;
#7668=CARTESIAN_POINT ( 'NONE',  ( 26.01652455409633902, -4.902371455920926380, -5.783357778048663356 ) ) ;
#7670=CARTESIAN_POINT ( 'NONE',  ( 29.52399153675929355, -1.971908820246954130, -5.783357778048658027 ) ) ;
#7672=CARTESIAN_POINT ( 'NONE',  ( 41.90164972253718645, -2.988527579590353422, -5.783357778048662468 ) ) ;
#7676=CARTESIAN_POINT ( 'NONE',  ( 27.12505156253147476, -7.276697974355294640, -5.783357778048668685 ) ) ;
#7681=EDGE_LOOP ( 'NONE', ( #7509, #2520 ) ) ;
#7685=CARTESIAN_POINT ( 'NONE',  ( 31.30154412293507349, -3.011689903141150815, -7.939653947423660263 ) ) ;
#7689=CARTESIAN_POINT ( 'NONE',  ( 27.12505156253147476, -7.276697974355294640, -5.783357778048668685 ) ) ;
#7691=EDGE_CURVE ( 'NONE', #17723, #16561, #11988, .T. ) ;
#7700=CARTESIAN_POINT ( 'NONE',  ( 29.30958546476020743, -4.505622649006972402, -8.283357778048662468 ) ) ;
#7702=CARTESIAN_POINT ( 'NONE',  ( 28.51709679197739078, -3.347160818026084339, -3.627061608673662008 ) ) ;
#7704=CARTESIAN_POINT ( 'NONE',  ( 27.29814976067589072, -3.294147343736874234, -8.283357778048660691 ) ) ;
#7708=ORIENTED_EDGE ( 'NONE', *, *, #7071, .F. ) ;
#7711=CARTESIAN_POINT ( 'NONE',  ( 32.04575515724927470, -1.668086104879473730, -5.783357778048658915 ) ) ;
#7715=DIRECTION ( 'NONE',  ( 0.1196152422706618645, -0.9928203230275510771, 0.000000000000000000 ) ) ;
#7723=CARTESIAN_POINT ( 'NONE',  ( 33.52375369703867847, -2.544085015380856518, -8.283357778048660691 ) ) ;
#7728=CARTESIAN_POINT ( 'NONE',  ( 26.00079723459025871, -4.771832887959356562, -3.592817407220987747 ) ) ;
#7731=CARTESIAN_POINT ( 'NONE',  ( 29.54600080245929306, -4.477139269648729325, -3.283357778048664688 ) ) ;
#7735=ADVANCED_FACE ( 'NONE', ( #16297 ), #9377, .T. ) ;
#7738=CARTESIAN_POINT ( 'NONE',  ( 26.92924972366625980, -7.310485091653801781, -5.783357778048657138 ) ) ;
#7749=CARTESIAN_POINT ( 'NONE',  ( 31.03886041246737548, -3.043338102658604161, -3.627061608673662008 ) ) ;
#7750=EDGE_CURVE ( 'NONE', #13433, #2203, #5292, .T. ) ;
#7760=ORIENTED_EDGE ( 'NONE', *, *, #4408, .F. ) ;
#7761=CARTESIAN_POINT ( 'NONE',  ( 25.71748644841968456, -2.420320648352046078, -5.783357778048663356 ) ) ;
#7767=FACE_OUTER_BOUND ( 'NONE', #778, .T. ) ;
#7770=CARTESIAN_POINT ( 'NONE',  ( 32.54050588463559990, -2.235448945602741766, -6.861505862736159145 ) ) ;
#7773=CARTESIAN_POINT ( 'NONE',  ( 27.30005507882132676, -4.747731375419166788, -3.627061608673664672 ) ) ;
#7788=CARTESIAN_POINT ( 'NONE',  ( 33.76207435632690590, -3.969185667289998332, -3.627061608673664672 ) ) ;
#7791=CARTESIAN_POINT ( 'NONE',  ( 28.40332666278570173, -4.614808937445885384, -7.939653947423662039 ) ) ;
#7794=CARTESIAN_POINT ( 'NONE',  ( 32.46178999037268653, -4.125844254797621957, -8.283357778048662468 ) ) ;
#7801=CARTESIAN_POINT ( 'NONE',  ( 32.50119254608192421, -4.121097024973739309, -3.627061608673664672 ) ) ;
#7823=CARTESIAN_POINT ( 'NONE',  ( 33.76397967447234549, -5.422769698972272678, -8.283357778048664244 ) ) ;
#7824=CARTESIAN_POINT ( 'NONE',  ( 27.38828526237195504, -6.917821758047558056, -4.533357778048668685 ) ) ;
#7825=CARTESIAN_POINT ( 'NONE',  ( 31.28415083292585663, -5.521667582366822202, -3.627061608673667781 ) ) ;
#7827=ORIENTED_EDGE ( 'NONE', *, *, #11232, .F. ) ;
#7847=CARTESIAN_POINT ( 'NONE',  ( 29.56783163384821833, -3.220568019956291383, -7.939653947423660263 ) ) ;
#7848=CARTESIAN_POINT ( 'NONE',  ( 33.28924367748503244, -4.026152426421394814, -7.939653947423662039 ) ) ;
#7855=CARTESIAN_POINT ( 'NONE',  ( 27.21934464581372737, -3.303641803799556964, -8.283357778048660691 ) ) ;
#7857=AXIS2_PLACEMENT_3D ( 'NONE', #6534, #9417, #7715 ) ;
#7864=CARTESIAN_POINT ( 'NONE',  ( 32.77709966008947617, -5.968767264923789284, -6.861505862736166250 ) ) ;
#7873=VERTEX_POINT ( 'NONE', #12726 ) ;
#7874=ORIENTED_EDGE ( 'NONE', *, *, #7106, .F. ) ;
#7876=CIRCLE ( 'NONE', #7595, 1.000000000000000000 ) ;
#7881=DIRECTION ( 'NONE',  ( -0.6674414130531752809, 0.7446623128248003320, -9.100287414781897985E-16 ) ) ;
#7884=CARTESIAN_POINT ( 'NONE',  ( 29.80442540930208750, -6.953886339277345563, -5.783357778048669573 ) ) ;
#7893=CARTESIAN_POINT ( 'NONE',  ( 33.32855701603872234, -2.140504347050403045, -6.861505862736158257 ) ) ;
#7912=CARTESIAN_POINT ( 'NONE',  ( 39.19942832275109623, -5.640193629429878897, -9.783357778048662468 ) ) ;
#7914=CARTESIAN_POINT ( 'NONE',  ( 30.78070346053490880, -6.209293581256383199, -4.705209693361168455 ) ) ;
#7924=DIRECTION ( 'NONE',  ( 0.1196152422706596996, -0.9928203230275514102, 0.000000000000000000 ) ) ;
#7929=DIRECTION ( 'NONE',  ( 5.615616396709274052E-18, -4.661026453772598353E-17, -1.000000000000000000 ) ) ;
#7934=CARTESIAN_POINT ( 'NONE',  ( 29.55043834383899437, -5.730545699181964991, -3.627061608673668225 ) ) ;
#7937=EDGE_LOOP ( 'NONE', ( #9437, #6048, #10634, #11925 ) ) ;
#7962=ORIENTED_EDGE ( 'NONE', *, *, #5877, .F. ) ;
#7969=CARTESIAN_POINT ( 'NONE',  ( 30.09392748191118017, -6.591845302810410701, -7.033357778048666908 ) ) ;
#7971=CARTESIAN_POINT ( 'NONE',  ( 27.88665588685489993, -3.423116496867954162, -3.627061608673662008 ) ) ;
#7973=CARTESIAN_POINT ( 'NONE',  ( 31.67744797322171735, -2.039621600994187656, -7.033357778048658027 ) ) ;
#7978=CARTESIAN_POINT ( 'NONE',  ( 33.58707084003705745, -6.498152266226124851, -5.783357778048669573 ) ) ;
#7981=EDGE_CURVE ( 'NONE', #3342, #7401, #8593, .T. ) ;
#7999=CARTESIAN_POINT ( 'NONE',  ( 32.02836186724004364, -4.178063784105134459, -7.939653947423662039 ) ) ;
#8000=CARTESIAN_POINT ( 'NONE',  ( 39.19942832275109623, -5.640193629429882449, -2.283357778048670461 ) ) ;
#8002=ORIENTED_EDGE ( 'NONE', *, *, #8443, .F. ) ;
#8005=ADVANCED_FACE ( 'NONE', ( #3584 ), #586, .T. ) ;
#8007=ORIENTED_EDGE ( 'NONE', *, *, #16942, .T. ) ;
#8011=CARTESIAN_POINT ( 'NONE',  ( 26.49878054387835746, -2.963357534503999968, -4.705209693361160461 ) ) ;
#8013=ADVANCED_FACE ( 'NONE', ( #4153 ), #9398, .T. ) ;
#8028=PRODUCT_DEFINITION_FORMATION_WITH_SPECIFIED_SOURCE ( 'ANY', '', #6352, .NOT_KNOWN. ) ;
#8030=CARTESIAN_POINT ( 'NONE',  ( 27.93543013035303701, -2.153102235610331316, -5.113484796970857893 ) ) ;
#8050=CARTESIAN_POINT ( 'NONE',  ( 28.52162355051263987, -6.481468097106410475, -6.861505862736167138 ) ) ;
#8052=CARTESIAN_POINT ( 'NONE',  ( 33.24613200752366282, -6.212066908601060256, -7.033357778048666908 ) ) ;
#8054=DIRECTION ( 'NONE',  ( 0.9928203230275512992, 0.1196152422706610180, 4.006172263299093133E-17 ) ) ;
#8057=( NAMED_UNIT ( * ) PLANE_ANGLE_UNIT ( ) SI_UNIT ( $, .RADIAN. ) );
#8060=EDGE_CURVE ( 'NONE', #4820, #16771, #10479, .T. ) ;
#8061=CARTESIAN_POINT ( 'NONE',  ( 27.78610916120306129, -6.570083055755264745, -4.705209693361169343 ) ) ;
#8072=CARTESIAN_POINT ( 'NONE',  ( 28.74176732417158320, -7.092112515190875044, -5.783357778048657138 ) ) ;
#8084=CYLINDRICAL_SURFACE ( 'NONE', #8759, 2.500000000000001776 ) ;
#8086=CARTESIAN_POINT ( 'NONE',  ( 26.86291784143654127, -6.981118157082444320, -7.033357778048666908 ) ) ;
#8087=CARTESIAN_POINT ( 'NONE',  ( 32.75517961154501023, -5.344437665069116328, -7.939653947423662927 ) ) ;
#8089=EDGE_CURVE ( 'NONE', #17584, #15376, #11273, .T. ) ;
#8102=CARTESIAN_POINT ( 'NONE',  ( 25.78518620311324838, -3.676302093007511651, -7.939653947423660263 ) ) ;
#8109=CARTESIAN_POINT ( 'NONE',  ( 39.42387297280458114, -7.503110141889759888, -6.033357778048665132 ) ) ;
#8115=VERTEX_POINT ( 'NONE', #4052 ) ;
#8146=CARTESIAN_POINT ( 'NONE',  ( 26.24443550082169807, -6.794058631016747896, -7.409555870055547722 ) ) ;
#8147=CARTESIAN_POINT ( 'NONE',  ( 28.72797218747911074, -6.756415940301135237, -4.533357778048668685 ) ) ;
#8154=CARTESIAN_POINT ( 'NONE',  ( 28.93739072872572393, -3.296523698798161650, -7.939653947423660263 ) ) ;
#8155=AXIS2_PLACEMENT_3D ( 'NONE', #13025, #7336, #9932 ) ;
#8167=CARTESIAN_POINT ( 'NONE',  ( 30.01874226414561875, -2.539271660970221944, -6.861505862736159145 ) ) ;
#8176=AXIS2_PLACEMENT_3D ( 'NONE', #8394, #1071, #14939 ) ;
#8181=CARTESIAN_POINT ( 'NONE',  ( 30.25080928106424594, -3.138282701210941994, -3.627061608673662896 ) ) ;
#8185=ADVANCED_FACE ( 'NONE', ( #11465 ), #4585, .T. ) ;
#8186=CARTESIAN_POINT ( 'NONE',  ( 32.58190297908952004, -5.565186596593329149, -8.283357778048664244 ) ) ;
#8198=CARTESIAN_POINT ( 'NONE',  ( 25.96860978910007844, -6.167287525404733017, -7.540302725459484989 ) ) ;
#8203=CARTESIAN_POINT ( 'NONE',  ( 38.92318875345451090, -3.347373306402334769, -5.783357778048662468 ) ) ;
#8207=ORIENTED_EDGE ( 'NONE', *, *, #13177, .F. ) ;
#8212=ADVANCED_FACE ( 'NONE', ( #14202 ), #9898, .T. ) ;
#8214=CARTESIAN_POINT ( 'NONE',  ( 31.05948030073166066, -1.776715885202022394, -5.783357778048661579 ) ) ;
#8220=LINE ( 'NONE', #2600, #14533 ) ;
#8232=CARTESIAN_POINT ( 'NONE',  ( 29.81991338116587542, -2.990324628369393611, -8.283357778048658915 ) ) ;
#8238=( NAMED_UNIT ( * ) SI_UNIT ( $, .STERADIAN. ) SOLID_ANGLE_UNIT ( ) );
#8240=CARTESIAN_POINT ( 'NONE',  ( 30.29464937815318493, -4.386941900920275472, -7.939653947423662039 ) ) ;
#8251=CARTESIAN_POINT ( 'NONE',  ( 28.34209327568754233, -5.876127416962207306, -7.939653947423664704 ) ) ;
#8253=CARTESIAN_POINT ( 'NONE',  ( 41.90164972253718645, -2.988527579590353422, -5.783357778048662468 ) ) ;
#8259=DIRECTION ( 'NONE',  ( 0.9928203230275510771, 0.1196152422706609902, 4.006172263299092517E-17 ) ) ;
#8263=CARTESIAN_POINT ( 'NONE',  ( 30.25533603959949502, -6.272589980291270351, -6.861505862736166250 ) ) ;
#8264=EDGE_LOOP ( 'NONE', ( #7122, #6879, #11445, #14602 ) ) ;
#8269=VERTEX_POINT ( 'NONE', #7144 ) ;
#8276=CARTESIAN_POINT ( 'NONE',  ( 27.77288575766320378, -4.690764616287755651, -7.939653947423662039 ) ) ;
#8278=ADVANCED_FACE ( 'NONE', ( #5850 ), #1834, .T. ) ;
#8283=DIRECTION ( 'NONE',  ( -0.7403740928408700794, 0.6721950629468047556, -3.769102058307143718E-16 ) ) ;
#8289=DIRECTION ( 'NONE',  ( -0.1196152422706610735, 0.9928203230275511881, 0.000000000000000000 ) ) ;
#8294=CARTESIAN_POINT ( 'NONE',  ( 27.99987602667382802, -2.482696394238434578, -4.533357778048659803 ) ) ;
#8299=FACE_OUTER_BOUND ( 'NONE', #16743, .T. ) ;
#8306=DIRECTION ( 'NONE',  ( -0.05980762113533058533, 0.4964101615137755386, 0.8660254037844385966 ) ) ;
#8307=ORIENTED_EDGE ( 'NONE', *, *, #10304, .T. ) ;
#8312=CARTESIAN_POINT ( 'NONE',  ( 27.28266178881210280, -7.257709054644824853, -5.783357778048669573 ) ) ;
#8314=CARTESIAN_POINT ( 'NONE',  ( 31.24973580796908834, -6.452593224933654170, -4.533357778048668685 ) ) ;
#8321=CARTESIAN_POINT ( 'NONE',  ( 28.40332666278570173, -4.614808937445885384, -7.939653947423662039 ) ) ;
#8323=DIRECTION ( 'NONE',  ( -0.9928203230275512992, -0.1196152422706610319, -9.614813431917826478E-17 ) ) ;
#8325=ORIENTED_EDGE ( 'NONE', *, *, #2157, .T. ) ;
#8328=DIRECTION ( 'NONE',  ( 0.9928203230275511881, 0.1196152422706610735, 9.614813431917827710E-17 ) ) ;
#8330=CARTESIAN_POINT ( 'NONE',  ( 32.50309786422735669, -5.574681056656013212, -8.283357778048664244 ) ) ;
#8332=CARTESIAN_POINT ( 'NONE',  ( 30.90769699326644826, -6.820963901304073929, -5.783357778048668685 ) ) ;
#8339=VERTEX_POINT ( 'NONE', #781 ) ;
#8345=CARTESIAN_POINT ( 'NONE',  ( 34.23532670761333918, -6.238269840783189579, -1.783357778048662690 ) ) ;
#8346=CARTESIAN_POINT ( 'NONE',  ( 30.80688261270428541, -4.325227911964988792, -3.283357778048664688 ) ) ;
#8348=CARTESIAN_POINT ( 'NONE',  ( 30.02326902268086428, -5.673578940050561847, -3.627061608673667781 ) ) ;
#8349=ORIENTED_EDGE ( 'NONE', *, *, #10304, .F. ) ;
#8363=CARTESIAN_POINT ( 'NONE',  ( 27.02867472334902033, -6.034368414549446058, -3.627061608673668225 ) ) ;
#8383=CARTESIAN_POINT ( 'NONE',  ( 33.40745134805642635, -4.011910736534825439, -3.283357778048664688 ) ) ;
#8394=CARTESIAN_POINT ( 'NONE',  ( 38.92318875345451090, -3.347373306402334769, -5.783357778048662468 ) ) ;
#8401=DIRECTION ( 'NONE',  ( 0.9928203230275510771, 0.1196152422706609902, 4.006172263299092517E-17 ) ) ;
#8404=CARTESIAN_POINT ( 'NONE',  ( 26.31556265977298992, -7.384422263489805793, -5.783357778048663356 ) ) ;
#8406=CARTESIAN_POINT ( 'NONE',  ( 30.88568772756644520, -4.315733451902305617, -3.283357778048664688 ) ) ;
#8410=CARTESIAN_POINT ( 'NONE',  ( 30.15026255541241440, -6.285249260098253465, -4.705209693361168455 ) ) ;
#8412=CARTESIAN_POINT ( 'NONE',  ( 29.17398450417959310, -7.029842018119214941, -5.783357778048669573 ) ) ;
#8422=DIRECTION ( 'NONE',  ( 0.1196152422706590474, -0.9928203230275514102, 0.000000000000000000 ) ) ;
#8425=CARTESIAN_POINT ( 'NONE',  ( 30.25533603959949502, -6.272589980291270351, -6.861505862736166250 ) ) ;
#8429=CARTESIAN_POINT ( 'NONE',  ( 27.27683486999669427, -2.232449958253242883, -5.783357778048658027 ) ) ;
#8435=LINE ( 'NONE', #15156, #44 ) ;
#8436=DIRECTION ( 'NONE',  ( 0.9928203230275510771, 0.1196152422706609902, 4.006172263299092517E-17 ) ) ;
#8439=CARTESIAN_POINT ( 'NONE',  ( 30.58169613980036772, -2.898544849976259385, -3.283357778048662023 ) ) ;
#8441=CARTESIAN_POINT ( 'NONE',  ( 27.75549246765397271, -7.200742295513424374, -5.783357778048668685 ) ) ;
#8443=EDGE_CURVE ( 'NONE', #15077, #14372, #967, .T. ) ;
#8450=EDGE_LOOP ( 'NONE', ( #6281, #3158, #3305, #12359 ) ) ;
#8455=ORIENTED_EDGE ( 'NONE', *, *, #15520, .T. ) ;
#8460=DIRECTION ( 'NONE',  ( -0.9928203230275510771, -0.1196152422706609902, -9.614813431917821547E-17 ) ) ;
#8461=CARTESIAN_POINT ( 'NONE',  ( 41.48299637458987377, 0.4863435510060803435, -5.783357778048662468 ) ) ;
#8464=CARTESIAN_POINT ( 'NONE',  ( 31.75254397038802878, -4.211294393702175398, -8.283357778048662468 ) ) ;
#8488=ORIENTED_EDGE ( 'NONE', *, *, #16754, .T. ) ;
#8499=CARTESIAN_POINT ( 'NONE',  ( 25.88156304229571703, -4.918631652813365562, -7.939653947423662039 ) ) ;
#8502=CARTESIAN_POINT ( 'NONE',  ( 29.30958546476020743, -4.505622649006972402, -8.283357778048662468 ) ) ;
#8504=LINE ( 'NONE', #4687, #15340 ) ;
#8505=CARTESIAN_POINT ( 'NONE',  ( 30.88125018618674744, -3.062327022369072171, -3.627061608673662896 ) ) ;
#8508=CARTESIAN_POINT ( 'NONE',  ( 26.01345249736710841, -4.876873030332669501, -8.181274557237335543 ) ) ;
#8512=EDGE_CURVE ( 'NONE', #16561, #12534, #7133, .T. ) ;
#8519=LINE ( 'NONE', #1640, #1206 ) ;
#8520=CARTESIAN_POINT ( 'NONE',  ( 30.78070346053490880, -6.209293581256383199, -4.705209693361168455 ) ) ;
#8521=CARTESIAN_POINT ( 'NONE',  ( 29.62480591732145996, -4.467644809586046151, -3.283357778048664688 ) ) ;
#8522=DIRECTION ( 'NONE',  ( -0.1196152422706610041, 0.9928203230275510771, 0.000000000000000000 ) ) ;
#8550=CARTESIAN_POINT ( 'NONE',  ( 33.06225340847440464, -6.234220648470727433, -4.533357778048668685 ) ) ;
#8559=PRESENTATION_STYLE_ASSIGNMENT (( #9905 ) ) ;
#8568=CARTESIAN_POINT ( 'NONE',  ( 33.35047706458318828, -2.764833946905071560, -7.939653947423660263 ) ) ;
#8574=EDGE_CURVE ( 'NONE', #6239, #6149, #16856, .T. ) ;
#8581=CARTESIAN_POINT ( 'NONE',  ( 46.37688276194213444, -2.449350377220338881, -5.783357778048662468 ) ) ;
#8585=CARTESIAN_POINT ( 'NONE',  ( 28.20260476654369697, -6.819712339336020612, -7.033357778048666908 ) ) ;
#8590=CARTESIAN_POINT ( 'NONE',  ( 31.28415083292585663, -5.521667582366822202, -3.627061608673667781 ) ) ;
#8591=CARTESIAN_POINT ( 'NONE',  ( 26.41562710823574278, -3.600346414165641828, -7.939653947423660263 ) ) ;
#8593=B_SPLINE_CURVE_WITH_KNOTS ( 'NONE', 3,
 ( #17202, #11810, #17389, #16009, #4745, #4922, #8923, #2143, #2044, #11721, #15910, #7570, #2228, #13097, #17291, #10450 ),
 .UNSPECIFIED., .F., .F.,
 ( 4, 2, 2, 2, 2, 2, 2, 4 ),
 ( 0.000000000000000000, 0.0008414457502979328513, 0.001262168625446899277, 0.001682891500595865703, 0.002103614375744832128, 0.002524337250893798554, 0.002945060126042764979, 0.003365783001191731405 ),
 .UNSPECIFIED. ) ;
#8597=ORIENTED_EDGE ( 'NONE', *, *, #15378, .T. ) ;
#8601=FACE_OUTER_BOUND ( 'NONE', #2441, .T. ) ;
#8603=EDGE_CURVE ( 'NONE', #15926, #6798, #15250, .T. ) ;
#8606=CARTESIAN_POINT ( 'NONE',  ( 32.04575515724926760, -1.668086104879473730, -5.783357778048658027 ) ) ;
#8608=LINE ( 'NONE', #5789, #12184 ) ;
#8614=CARTESIAN_POINT ( 'NONE',  ( 31.31418170428987224, -6.782187383561751659, -5.113484796970860558 ) ) ;
#8621=FACE_OUTER_BOUND ( 'NONE', #7127, .T. ) ;
#8638=LINE ( 'NONE', #663, #13252 ) ;
#8640=CARTESIAN_POINT ( 'NONE',  ( 33.10345976029034176, -2.594722134608779207, -3.283357778048662023 ) ) ;
#8642=CARTESIAN_POINT ( 'NONE',  ( 29.11066736118121767, -3.075774767273946608, -8.283357778048660691 ) ) ;
#8643=ORIENTED_EDGE ( 'NONE', *, *, #15743, .T. ) ;
#8645=VECTOR ( 'NONE', #4036, 1000.000000000000227 ) ;
#8658=CARTESIAN_POINT ( 'NONE',  ( 29.71979337562451207, -1.938121702948446323, -5.783357778048664244 ) ) ;
#8665=CARTESIAN_POINT ( 'NONE',  ( 33.21234388421201800, -5.489230917751459771, -8.283357778048664244 ) ) ;
#8673=CARTESIAN_POINT ( 'NONE',  ( 26.99805802979993885, -6.665027654307603022, -4.705209693361168455 ) ) ;
#8678=CARTESIAN_POINT ( 'NONE',  ( 26.01652455409633902, -4.902371455920926380, -5.783357778048663356 ) ) ;
#8687=CARTESIAN_POINT ( 'NONE',  ( 26.97551107961034944, -7.694459687869362519, -5.783357778048669573 ) ) ;
#8690=CARTESIAN_POINT ( 'NONE',  ( 30.88577694472199298, -6.196634301449400084, -6.861505862736166250 ) ) ;
#8694=CARTESIAN_POINT ( 'NONE',  ( 26.52522735095806894, -6.721994413439005278, -4.705209693361169343 ) ) ;
#8700=DIRECTION ( 'NONE',  ( 0.9928203230275511881, 0.1196152422706609764, 1.201851678989727817E-16 ) ) ;
#8705=CARTESIAN_POINT ( 'NONE',  ( 32.72003615946069743, -2.840789625746940938, -7.939653947423660263 ) ) ;
#8707=CYLINDRICAL_SURFACE ( 'NONE', #5226, 2.500000000000000000 ) ;
#8712=ORIENTED_EDGE ( 'NONE', *, *, #2478, .T. ) ;
#8721=DIRECTION ( 'NONE',  ( 0.9928203230275512992, 0.1196152422706610180, 4.006172263299093133E-17 ) ) ;
#8722=ORIENTED_EDGE ( 'NONE', *, *, #3576, .F. ) ;
#8724=AXIS2_PLACEMENT_3D ( 'NONE', #3818, #14704, #12049 ) ;
#8728=ORIENTED_EDGE ( 'NONE', *, *, #10540, .T. ) ;
#8732=EDGE_LOOP ( 'NONE', ( #6176, #1679, #14756, #13160, #6759, #5871 ) ) ;
#8740=CARTESIAN_POINT ( 'NONE',  ( 32.06776442294927421, -4.173316554281249147, -3.283357778048664688 ) ) ;
#8742=CARTESIAN_POINT ( 'NONE',  ( 29.40036258452792950, -7.012764792547963033, -6.453230759126474148 ) ) ;
#8759=AXIS2_PLACEMENT_3D ( 'NONE', #16611, #1560, #2649 ) ;
#8763=FACE_OUTER_BOUND ( 'NONE', #1521, .T. ) ;
#8764=CARTESIAN_POINT ( 'NONE',  ( 33.26181313012506280, -6.547536259434060923, -6.453230759126471483 ) ) ;
#8768=EDGE_LOOP ( 'NONE', ( #699, #10302, #14912, #2381 ) ) ;
#8770=CARTESIAN_POINT ( 'NONE',  ( 26.03917326857634151, -4.899642733102906433, -3.627061608673664672 ) ) ;
#8775=ORIENTED_EDGE ( 'NONE', *, *, #3042, .F. ) ;
#8780=( BOUNDED_CURVE ( )  B_SPLINE_CURVE ( 2, ( #15686, #4704, #4880, #7704, #7439, #15591, #17060, #14514, #6248 ),
 .UNSPECIFIED., .F., .T. ) 
 B_SPLINE_CURVE_WITH_KNOTS ( ( 3, 2, 2, 2, 3 ),
 ( 0.7115384615384615641, 0.7179487179487179516, 0.7307692307692307265, 0.7435897435897436125, 0.7500000000000000000 ),
 .UNSPECIFIED. ) 
 CURVE ( )  GEOMETRIC_REPRESENTATION_ITEM ( )  RATIONAL_B_SPLINE_CURVE ( ( 0.9330127018922194093, 0.9330127018922194093, 1.000000000000000000, 0.8660254037844387076, 1.000000000000000000, 0.8660254037844387076, 1.000000000000000000, 0.9330127018922194093, 0.9330127018922194093 ) ) 
 REPRESENTATION_ITEM ( '' )  );
#8781=CARTESIAN_POINT ( 'NONE',  ( 33.40754056521197413, -5.892811586081919906, -6.861505862736166250 ) ) ;
#8785=CARTESIAN_POINT ( 'NONE',  ( 32.65880277236253448, -4.102108105263264193, -7.939653947423662039 ) ) ;
#8787=EDGE_CURVE ( 'NONE', #5290, #17723, #17601, .T. ) ;
#8792=ORIENTED_EDGE ( 'NONE', *, *, #17495, .F. ) ;
#8800=CARTESIAN_POINT ( 'NONE',  ( 25.58373587974369201, -2.446631813008643075, -5.783357778048658027 ) ) ;
#8822=CARTESIAN_POINT ( 'NONE',  ( 26.86291784143654127, -6.981118157082444320, -7.033357778048666908 ) ) ;
#8828=CARTESIAN_POINT ( 'NONE',  ( 31.63243098167119172, -2.771952051906466874, -8.283357778048658915 ) ) ;
#8829=CARTESIAN_POINT ( 'NONE',  ( 29.06119811526816576, -2.017469425591354337, -6.453230759126464378 ) ) ;
#8845=CARTESIAN_POINT ( 'NONE',  ( 32.67619606237177265, -1.592130426037603907, -5.783357778048658027 ) ) ;
#8852=DIRECTION ( 'NONE',  ( -0.05980762113533193841, 0.4964101615137754275, 0.8660254037844385966 ) ) ;
#8853=VERTEX_POINT ( 'NONE', #2278 ) ;
#8865=CARTESIAN_POINT ( 'NONE',  ( 33.40301380667672504, -2.758504307001591549, -3.627061608673662896 ) ) ;
#8869=CARTESIAN_POINT ( 'NONE',  ( 27.50150540219088313, -5.977401655418042914, -3.627061608673667781 ) ) ;
#8871=CARTESIAN_POINT ( 'NONE',  ( 26.39370705969127684, -2.976016814310973313, -6.861505862736158257 ) ) ;
#8874=ORIENTED_EDGE ( 'NONE', *, *, #2408, .T. ) ;
#8880=CARTESIAN_POINT ( 'NONE',  ( 27.82847066025702887, -2.165988739474055791, -5.783357778048658027 ) ) ;
#8884=CARTESIAN_POINT ( 'NONE',  ( 32.70264286945147347, -5.350767304972614546, -3.627061608673668225 ) ) ;
#8889=CARTESIAN_POINT ( 'NONE',  ( 27.96989853965305528, -4.667028466753395222, -8.283357778048662468 ) ) ;
#8905=CARTESIAN_POINT ( 'NONE',  ( 39.85968403307006014, -4.832501846690662184, -8.531230242176626177 ) ) ;
#8909=CIRCLE ( 'NONE', #2270, 2.500000000000001776 ) ;
#8912=CARTESIAN_POINT ( 'NONE',  ( 31.34233605952372415, -6.778795339760710803, -5.783357778048663356 ) ) ;
#8914=CARTESIAN_POINT ( 'NONE',  ( 29.38468146192651886, -6.677295441714964142, -7.033357778048666908 ) ) ;
#8921=ORIENTED_EDGE ( 'NONE', *, *, #13725, .T. ) ;
#8923=CARTESIAN_POINT ( 'NONE',  ( 25.78902048130849067, -3.014061381488925218, -4.757751673912568258 ) ) ;
#8930=CARTESIAN_POINT ( 'NONE',  ( 29.13014440709066832, -5.781182818409868140, -7.939653947423664704 ) ) ;
#8933=VECTOR ( 'NONE', #13306, 1000.000000000000227 ) ;
#8938=CARTESIAN_POINT ( 'NONE',  ( 25.72395281601508898, -4.937620572523835349, -7.939653947423662039 ) ) ;
#8942=CARTESIAN_POINT ( 'NONE',  ( 41.91396146090167463, 0.4627762229654553972, -5.783357778048662468 ) ) ;
#8944=ORIENTED_EDGE ( 'NONE', *, *, #2539, .F. ) ;
#8948=CARTESIAN_POINT ( 'NONE',  ( 26.31046454879147944, -7.342107353655505264, -6.247327665911178052 ) ) ;
#8950=ORIENTED_EDGE ( 'NONE', *, *, #829, .T. ) ;
#8951=CARTESIAN_POINT ( 'NONE',  ( 26.31128205117621022, -7.047579375861630524, -7.033357778048666908 ) ) ;
#8954=CARTESIAN_POINT ( 'NONE',  ( 26.23609683341064525, -2.995005734021441768, -6.861505862736159145 ) ) ;
#8955=CARTESIAN_POINT ( 'NONE',  ( 33.12669930479518854, -6.563814807098823145, -5.113484796970860558 ) ) ;
#8957=VECTOR ( 'NONE', #14315, 1000.000000000000114 ) ;
#8960=ORIENTED_EDGE ( 'NONE', *, *, #7640, .T. ) ;
#8969=CARTESIAN_POINT ( 'NONE',  ( 26.36761712467744090, -6.740983333149474177, -4.705209693361168455 ) ) ;
#8974=CARTESIAN_POINT ( 'NONE',  ( 26.87785582392756112, -3.344784462964796035, -3.283357778048662023 ) ) ;
#8977=ORIENTED_EDGE ( 'NONE', *, *, #4806, .T. ) ;
#8980=CARTESIAN_POINT ( 'NONE',  ( 32.28234893270314387, -5.401404424200516807, -7.939653947423662927 ) ) ;
#8981=ORIENTED_EDGE ( 'NONE', *, *, #15378, .F. ) ;
#8990=ORIENTED_EDGE ( 'NONE', *, *, #17495, .T. ) ;
#9002=CARTESIAN_POINT ( 'NONE',  ( 26.79905070906540132, -3.354278923027479209, -3.283357778048662023 ) ) ;
#9004=FACE_OUTER_BOUND ( 'NONE', #13946, .T. ) ;
#9008=DIRECTION ( 'NONE',  ( 0.9928203230275512992, 0.1196152422706610180, 4.006172263299093133E-17 ) ) ;
#9023=DIRECTION ( 'NONE',  ( -0.1196152422706610735, 0.9928203230275511881, 0.000000000000000000 ) ) ;
#9024=CARTESIAN_POINT ( 'NONE',  ( 28.51709679197739078, -3.347160818026084339, -3.627061608673662008 ) ) ;
#9031=CARTESIAN_POINT ( 'NONE',  ( 26.23609683341064525, -2.995005734021441768, -6.861505862736159145 ) ) ;
#9034=CARTESIAN_POINT ( 'NONE',  ( 29.37220822929407760, -7.016156836349003001, -5.783357778048668685 ) ) ;
#9035=CARTESIAN_POINT ( 'NONE',  ( 27.49335874655903567, -6.905162478240574053, -7.033357778048666908 ) ) ;
#9042=CARTESIAN_POINT ( 'NONE',  ( 32.14665875496697822, -6.044722943765660439, -6.861505862736166250 ) ) ;
#9046=CARTESIAN_POINT ( 'NONE',  ( 28.73594040535616756, -2.066853418799292630, -5.783357778048658027 ) ) ;
#9062=CARTESIAN_POINT ( 'NONE',  ( 30.82871344409320713, -3.068656662272551738, -7.939653947423660263 ) ) ;
#9069=CARTESIAN_POINT ( 'NONE',  ( 27.10304229683147526, -4.771467524953526329, -3.283357778048664688 ) ) ;
#9075=CARTESIAN_POINT ( 'NONE',  ( 33.35047706458318828, -2.764833946905070672, -7.939653947423660263 ) ) ;
#9076=EDGE_LOOP ( 'NONE', ( #1576, #8007, #3330, #5196 ) ) ;
#9082=CARTESIAN_POINT ( 'NONE',  ( 32.55182397003001427, -2.661183353387966299, -3.283357778048662023 ) ) ;
#9086=CARTESIAN_POINT ( 'NONE',  ( 33.47428445112562656, -1.485779673698264913, -6.453230759126466154 ) ) ;
#9095=CARTESIAN_POINT ( 'NONE',  ( 29.91004888286193619, -6.613999042680076990, -4.533357778048668685 ) ) ;
#9096=CARTESIAN_POINT ( 'NONE',  ( 31.08270050955629671, -4.291997302367946077, -3.627061608673664672 ) ) ;
#9100=CARTESIAN_POINT ( 'NONE',  ( 30.03006034954003667, -2.965006068755446478, -3.283357778048662023 ) ) ;
#9110=( BOUNDED_CURVE ( )  B_SPLINE_CURVE ( 2, ( #425, #4401, #7134, #14103, #9916, #8665, #595, #8764, #3222 ),
 .UNSPECIFIED., .F., .T. ) 
 B_SPLINE_CURVE_WITH_KNOTS ( ( 3, 2, 2, 2, 3 ),
 ( 0.01923076923076924571, 0.02564102564102564014, 0.03846153846153846367, 0.05128205128205128027, 0.05769230769230770939 ),
 .UNSPECIFIED. ) 
 CURVE ( )  GEOMETRIC_REPRESENTATION_ITEM ( )  RATIONAL_B_SPLINE_CURVE ( ( 0.9330127018922194093, 0.9330127018922195203, 1.000000000000000000, 0.8660254037844387076, 1.000000000000000000, 0.8660254037844387076, 1.000000000000000000, 0.9330127018922191873, 0.9330127018922194093 ) ) 
 REPRESENTATION_ITEM ( '' )  );
#9115=DIRECTION ( 'NONE',  ( -0.1196152422706610735, 0.9928203230275511881, 0.000000000000000000 ) ) ;
#9116=CARTESIAN_POINT ( 'NONE',  ( 31.06530721954707985, -6.801974981593605030, -5.783357778048669573 ) ) ;
#9122=LINE ( 'NONE', #17833, #9890 ) ;
#9123=VERTEX_POINT ( 'NONE', #1898 ) ;
#9127=VERTEX_POINT ( 'NONE', #2982 ) ;
#9133=CARTESIAN_POINT ( 'NONE',  ( 31.27962407439061110, -2.387360303286481855, -6.861505862736159145 ) ) ;
#9137=CARTESIAN_POINT ( 'NONE',  ( 29.41022140756759029, -3.239556939666760726, -7.939653947423660263 ) ) ;
#9145=ORIENTED_EDGE ( 'NONE', *, *, #10273, .F. ) ;
#9150=DIRECTION ( 'NONE',  ( -0.9928203230275510771, -0.1196152422706614760, -0.000000000000000000 ) ) ;
#9152=CARTESIAN_POINT ( 'NONE',  ( 28.54354359905709870, -7.105797696961086096, -5.783357778048669573 ) ) ;
#9153=CARTESIAN_POINT ( 'NONE',  ( 30.63309003953906995, -6.864245478665264244, -5.783357778048663356 ) ) ;
#9161=CARTESIAN_POINT ( 'NONE',  ( 30.82871344409320713, -3.068656662272551294, -7.939653947423660263 ) ) ;
#9166=ORIENTED_EDGE ( 'NONE', *, *, #4667, .F. ) ;
#9178=CARTESIAN_POINT ( 'NONE',  ( 28.12379965168153362, -6.829206799398704675, -7.033357778048666908 ) ) ;
#9179=CARTESIAN_POINT ( 'NONE',  ( 32.04158527077989760, -6.057382223572642665, -4.705209693361168455 ) ) ;
#9186=( BOUNDED_CURVE ( )  B_SPLINE_CURVE ( 2, ( #10714, #14990, #5193, #6565, #2239, #12085, #862 ),
 .UNSPECIFIED., .F., .T. ) 
 B_SPLINE_CURVE_WITH_KNOTS ( ( 3, 2, 2, 3 ),
 ( 0.9423076923076922906, 0.9487179487179486781, 0.9615384615384615641, 0.9690340935984054216 ),
 .UNSPECIFIED. ) 
 CURVE ( )  GEOMETRIC_REPRESENTATION_ITEM ( )  RATIONAL_B_SPLINE_CURVE ( ( 0.9330127018922194093, 0.9330127018922194093, 1.000000000000000000, 0.8660254037844387076, 1.000000000000000000, 0.9216705062683109295, 0.9349331465915117212 ) ) 
 REPRESENTATION_ITEM ( '' )  );
#9196=CARTESIAN_POINT ( 'NONE',  ( 30.29464937815318493, -4.386941900920275472, -7.939653947423662039 ) ) ;
#9197=CARTESIAN_POINT ( 'NONE',  ( 28.82057243903374655, -7.082618055128190093, -5.783357778048668685 ) ) ;
#9211=CARTESIAN_POINT ( 'NONE',  ( 32.14213199643172914, -2.910415664685331638, -3.627061608673662896 ) ) ;
#9215=CARTESIAN_POINT ( 'NONE',  ( 32.00093131988006689, -6.699447617117800569, -6.453230759126470595 ) ) ;
#9217=CARTESIAN_POINT ( 'NONE',  ( 27.60205212784272177, -2.830435096530727446, -4.705209693361161349 ) ) ;
#9221=ORIENTED_EDGE ( 'NONE', *, *, #16269, .T. ) ;
#9224=ORIENTED_EDGE ( 'NONE', *, *, #1662, .T. ) ;
#9230=CARTESIAN_POINT ( 'NONE',  ( 30.29464937815318493, -4.386941900920275472, -7.939653947423662039 ) ) ;
#9232=CARTESIAN_POINT ( 'NONE',  ( 31.51612863268893960, -4.239777773060436239, -3.283357778048664688 ) ) ;
#9234=EDGE_CURVE ( 'NONE', #15769, #4820, #8504, .T. ) ;
#9241=CARTESIAN_POINT ( 'NONE',  ( 31.45915434921569798, -2.992700983430681028, -7.939653947423660263 ) ) ;
#9252=CARTESIAN_POINT ( 'NONE',  ( 28.28511899221430070, -4.629050627332469858, -3.283357778048664688 ) ) ;
#9258=EDGE_LOOP ( 'NONE', ( #9685, #4208, #3557, #6754 ) ) ;
#9262=CARTESIAN_POINT ( 'NONE',  ( 46.86575133767496482, -2.390451368237048513, -5.783357778048662468 ) ) ;
#9263=CARTESIAN_POINT ( 'NONE',  ( 29.04309111455793513, -1.630102785574754742, -5.783357778048658027 ) ) ;
#9264=AXIS2_PLACEMENT_3D ( 'NONE', #6408, #17226, #16123 ) ;
#9265=CARTESIAN_POINT ( 'NONE',  ( 32.12473870642251939, -5.420393343910986594, -7.939653947423662927 ) ) ;
#9272=DIRECTION ( 'NONE',  ( 1.000000000000000000, 0.000000000000000000, 0.000000000000000000 ) ) ;
#9284=CARTESIAN_POINT ( 'NONE',  ( 31.02146712245815507, -5.553315781884258229, -7.939653947423664704 ) ) ;
#9285=CARTESIAN_POINT ( 'NONE',  ( 33.40301380667672504, -2.758504307001591549, -3.627061608673662896 ) ) ;
#9309=VECTOR ( 'NONE', #1105, 1000.000000000000227 ) ;
#9321=CARTESIAN_POINT ( 'NONE',  ( 28.41655006632555569, -6.494127376913395366, -4.705209693361169343 ) ) ;
#9323=DIRECTION ( 'NONE',  ( 0.05980762113533041185, -0.4964101615137758161, 0.8660254037844385966 ) ) ;
#9326=CARTESIAN_POINT ( 'NONE',  ( 31.78252145740879797, -2.026962321187214311, -4.533357778048659803 ) ) ;
#9330=CARTESIAN_POINT ( 'NONE',  ( 33.56062403295735663, -2.739515387291123982, -3.627061608673662008 ) ) ;
#9331=ORIENTED_EDGE ( 'NONE', *, *, #12904, .F. ) ;
#9333=DIRECTION ( 'NONE',  ( -0.1196152422706609625, 0.9928203230275510771, 0.000000000000000000 ) ) ;
#9335=EDGE_LOOP ( 'NONE', ( #9977, #8944, #14682, #1300 ) ) ;
#9349=CARTESIAN_POINT ( 'NONE',  ( 26.27285561281999193, -7.029948842322393254, -4.710679390969556124 ) ) ;
#9352=CARTESIAN_POINT ( 'NONE',  ( 26.89670596474818609, -7.703954147932045693, -5.783357778048669573 ) ) ;
#9353=CARTESIAN_POINT ( 'NONE',  ( 32.65880277236253448, -4.102108105263264193, -7.939653947423662039 ) ) ;
#9366=CARTESIAN_POINT ( 'NONE',  ( 33.59503905791412137, -1.808589744724287129, -4.533357778048659803 ) ) ;
#9369=ORIENTED_EDGE ( 'NONE', *, *, #6043, .T. ) ;
#9371=ADVANCED_FACE ( 'NONE', ( #17319 ), #14494, .F. ) ;
#9377=CYLINDRICAL_SURFACE ( 'NONE', #13622, 2.500000000000001776 ) ;
#9393=ORIENTED_EDGE ( 'NONE', *, *, #11616, .F. ) ;
#9394=ORIENTED_EDGE ( 'NONE', *, *, #7691, .T. ) ;
#9395=EDGE_CURVE ( 'NONE', #10652, #17258, #1027, .T. ) ;
#9398=CYLINDRICAL_SURFACE ( 'NONE', #4696, 2.500000000000001776 ) ;
#9404=CARTESIAN_POINT ( 'NONE',  ( 28.91547068018125799, -2.672194098943493135, -6.861505862736158257 ) ) ;
#9407=CARTESIAN_POINT ( 'NONE',  ( 32.77701044293393551, -4.087866415376695706, -3.283357778048664688 ) ) ;
#9414=CARTESIAN_POINT ( 'NONE',  ( 29.78250536075762867, -6.329556739422670830, -6.861505862736167138 ) ) ;
#9417=DIRECTION ( 'NONE',  ( -0.9928203230275512992, -0.1196152422706610180, -4.006172263299093133E-17 ) ) ;
#9429=VERTEX_POINT ( 'NONE', #8214 ) ;
#9435=CARTESIAN_POINT ( 'NONE',  ( 32.77709966008947617, -5.968767264923789284, -6.861505862736166250 ) ) ;
#9437=ORIENTED_EDGE ( 'NONE', *, *, #7691, .F. ) ;
#9440=ORIENTED_EDGE ( 'NONE', *, *, #12115, .T. ) ;
#9447=EDGE_CURVE ( 'NONE', #15376, #16997, #2862, .T. ) ;
#9449=EDGE_CURVE ( 'NONE', #13433, #2702, #3872, .T. ) ;
#9452=CARTESIAN_POINT ( 'NONE',  ( 33.45617745041539592, -1.098413033681664430, -5.783357778048658027 ) ) ;
#9455=ORIENTED_EDGE ( 'NONE', *, *, #4408, .T. ) ;
#9456=CARTESIAN_POINT ( 'NONE',  ( 26.13613979636700080, -5.895191778948487560, -5.783357778048664244 ) ) ;
#9462=LINE ( 'NONE', #7761, #5274 ) ;
#9463=DIRECTION ( 'NONE',  ( 0.1196152422706590474, -0.9928203230275514102, 0.000000000000000000 ) ) ;
#9473=CARTESIAN_POINT ( 'NONE',  ( 26.01652455409633902, -4.902371455920926380, -5.783357778048663356 ) ) ;
#9485=CARTESIAN_POINT ( 'NONE',  ( 31.27600417729400917, -6.449428405189353342, -7.033357778048666908 ) ) ;
#9491=CARTESIAN_POINT ( 'NONE',  ( 28.13873763417254992, -3.192873105281056390, -3.283357778048662023 ) ) ;
#9498=CARTESIAN_POINT ( 'NONE',  ( 29.67743187657054449, -6.342216019229654833, -4.705209693361169343 ) ) ;
#9500=DIRECTION ( 'NONE',  ( -0.1196152422706611984, 0.9928203230275511881, 0.000000000000000000 ) ) ;
#9508=CARTESIAN_POINT ( 'NONE',  ( 28.25893984004492765, -6.513116296623863377, -4.705209693361168455 ) ) ;
#9520=CARTESIAN_POINT ( 'NONE',  ( 29.39282811755836988, -5.749534618892433002, -3.627061608673667781 ) ) ;
#9525=ORIENTED_EDGE ( 'NONE', *, *, #9618, .T. ) ;
#9538=CARTESIAN_POINT ( 'NONE',  ( 27.86926259684567597, -5.933094176093606897, -7.939653947423664704 ) ) ;
#9547=ORIENTED_EDGE ( 'NONE', *, *, #15251, .F. ) ;
#9572=CARTESIAN_POINT ( 'NONE',  ( 30.41656616297672500, -2.191532958677927745, -7.033357778048658027 ) ) ;
#9578=CARTESIAN_POINT ( 'NONE',  ( 27.00222791626931240, -2.275731535614434531, -5.783357778048658915 ) ) ;
#9582=CARTESIAN_POINT ( 'NONE',  ( 31.68992120585416217, -1.700760206360153015, -5.783357778048664244 ) ) ;
#9591=CARTESIAN_POINT ( 'NONE',  ( 28.99445422935450267, -6.424501337975009996, -6.861505862736166250 ) ) ;
#9593=PLANE ( 'NONE',  #14527 ) ;
#9604=CARTESIAN_POINT ( 'NONE',  ( 27.93049598394382116, -4.671775696577297410, -3.627061608673664672 ) ) ;
#9614=ORIENTED_EDGE ( 'NONE', *, *, #3519, .F. ) ;
#9615=VECTOR ( 'NONE', #12998, 1000.000000000000227 ) ;
#9618=EDGE_CURVE ( 'NONE', #12431, #15077, #2332, .T. ) ;
#9622=CARTESIAN_POINT ( 'NONE',  ( 25.71748644841968456, -2.420320648352046078, -5.783357778048663356 ) ) ;
#9623=CARTESIAN_POINT ( 'NONE',  ( 32.24155699611449677, -1.634298987580965923, -5.783357778048664244 ) ) ;
#9624=CARTESIAN_POINT ( 'NONE',  ( 27.25621498173240198, -3.499072175709823984, -3.627061608673662008 ) ) ;
#9639=VECTOR ( 'NONE', #10663, 1000.000000000000227 ) ;
#9643=( BOUNDED_CURVE ( )  B_SPLINE_CURVE ( 2, ( #15298, #16672, #5587, #2880, #7067, #4245, #76, #14538, #14438 ),
 .UNSPECIFIED., .F., .T. ) 
 B_SPLINE_CURVE_WITH_KNOTS ( ( 3, 2, 2, 2, 3 ),
 ( 0.2115384615384615641, 0.2179487179487179516, 0.2307692307692307820, 0.2435897435897435848, 0.2500000000000000000 ),
 .UNSPECIFIED. ) 
 CURVE ( )  GEOMETRIC_REPRESENTATION_ITEM ( )  RATIONAL_B_SPLINE_CURVE ( ( 0.9330127018922194093, 0.9330127018922196314, 1.000000000000000000, 0.8660254037844387076, 1.000000000000000000, 0.8660254037844387076, 1.000000000000000000, 0.9330127018922191873, 0.9330127018922194093 ) ) 
 REPRESENTATION_ITEM ( '' )  );
#9654=CARTESIAN_POINT ( 'NONE',  ( 31.24221605398236079, -5.726592414339752857, -8.283357778048664244 ) ) ;
#9659=CARTESIAN_POINT ( 'NONE',  ( 28.99436501219896201, -4.543600488427916417, -3.283357778048664688 ) ) ;
#9663=( LENGTH_UNIT ( ) NAMED_UNIT ( * ) SI_UNIT ( .MILLI., .METRE. ) );
#9665=( BOUNDED_CURVE ( )  B_SPLINE_CURVE ( 2, ( #7082, #15412, #9951, #13783, #15502, #14137, #2998, #11402, #4346 ),
 .UNSPECIFIED., .F., .T. ) 
 B_SPLINE_CURVE_WITH_KNOTS ( ( 3, 2, 2, 2, 3 ),
 ( 0.05769230769230771633, 0.06410256410256409687, 0.07692307692307692735, 0.08974358974358974395, 0.09615384615384617306 ),
 .UNSPECIFIED. ) 
 CURVE ( )  GEOMETRIC_REPRESENTATION_ITEM ( )  RATIONAL_B_SPLINE_CURVE ( ( 0.9330127018922194093, 0.9330127018922196314, 1.000000000000000000, 0.8660254037844387076, 1.000000000000000000, 0.8660254037844387076, 1.000000000000000000, 0.9330127018922191873, 0.9330127018922194093 ) ) 
 REPRESENTATION_ITEM ( '' )  );
#9668=CARTESIAN_POINT ( 'NONE',  ( 28.91999743871649997, -5.806501378023834370, -3.627061608673668225 ) ) ;
#9673=ORIENTED_EDGE ( 'NONE', *, *, #7981, .F. ) ;
#9679=CARTESIAN_POINT ( 'NONE',  ( 27.93049598394382116, -4.671775696577297410, -3.627061608673664672 ) ) ;
#9685=ORIENTED_EDGE ( 'NONE', *, *, #3693, .F. ) ;
#9692=CARTESIAN_POINT ( 'NONE',  ( 29.36638131047866906, -1.990897739957422807, -5.783357778048658915 ) ) ;
#9706=CARTESIAN_POINT ( 'NONE',  ( 26.63030083514515312, -6.709335133632020387, -6.861505862736167138 ) ) ;
#9715=EDGE_LOOP ( 'NONE', ( #17012, #2716, #13777, #11532, #9921, #17006, #2846, #8307, #6259, #2710, #5068, #6354, #15112, #7193, #15398, #4671, #9224, #5556, #3539, #17788, #15524, #8712, #10718, #9394, #454, #8921, #9369, #13037, #13764 ) ) ;
#9716=VERTEX_POINT ( 'NONE', #11540 ) ;
#9730=ORIENTED_EDGE ( 'NONE', *, *, #16806, .T. ) ;
#9737=FACE_OUTER_BOUND ( 'NONE', #17462, .T. ) ;
#9741=CARTESIAN_POINT ( 'NONE',  ( 25.74134610602432360, -2.427642893298174620, -5.783357778048658027 ) ) ;
#9742=CARTESIAN_POINT ( 'NONE',  ( 26.16860980394290337, -3.430234601869349920, -3.283357778048662023 ) ) ;
#9744=CARTESIAN_POINT ( 'NONE',  ( 28.83304567166618781, -6.743756660494150346, -7.033357778048666908 ) ) ;
#9750=CARTESIAN_POINT ( 'NONE',  ( 32.34358231980129261, -4.140085944684206432, -3.627061608673664672 ) ) ;
#9752=CARTESIAN_POINT ( 'NONE',  ( 29.65098506949083301, -2.583579140294649523, -4.705209693361160461 ) ) ;
#9762=CARTESIAN_POINT ( 'NONE',  ( 30.25080928106424594, -3.138282701210941994, -3.627061608673662896 ) ) ;
#9765=DIRECTION ( 'NONE',  ( 0.9928203230275511881, 0.1196152422706610180, 9.614813431917825245E-17 ) ) ;
#9776=CARTESIAN_POINT ( 'NONE',  ( 30.35023428074701002, -1.862166024106576057, -5.783357778048664244 ) ) ;
#9778=CARTESIAN_POINT ( 'NONE',  ( 29.99682221560115991, -1.914942061115552541, -5.783357778048658915 ) ) ;
#9794=ADVANCED_FACE ( 'NONE', ( #13191 ), #855, .T. ) ;
#9798=CARTESIAN_POINT ( 'NONE',  ( 32.89331279191618762, -2.620040694222726785, -8.283357778048658915 ) ) ;
#9807=CARTESIAN_POINT ( 'NONE',  ( 33.78529456515154550, -6.484467084455913799, -5.783357778048663356 ) ) ;
#9810=ORIENTED_EDGE ( 'NONE', *, *, #5877, .T. ) ;
#9811=VECTOR ( 'NONE', #9150, 1000.000000000000114 ) ;
#9821=CARTESIAN_POINT ( 'NONE',  ( 32.32618902979206865, -6.650063623909865385, -5.783357778048669573 ) ) ;
#9834=ORIENTED_EDGE ( 'NONE', *, *, #14225, .T. ) ;
#9837=DIRECTION ( 'NONE',  ( 0.6287809056569716448, 0.6925565483635240938, -0.3535533905932743415 ) ) ;
#9842=CARTESIAN_POINT ( 'NONE',  ( 30.57046727500519978, -4.353711291323232757, -8.283357778048662468 ) ) ;
#9845=CARTESIAN_POINT ( 'NONE',  ( 30.86385689617752348, -5.572304701594726239, -7.939653947423664704 ) ) ;
#9847=CARTESIAN_POINT ( 'NONE',  ( 25.90419076669538256, -3.969988049114259177, -7.913474645583921330 ) ) ;
#9852=ORIENTED_EDGE ( 'NONE', *, *, #5421, .F. ) ;
#9858=CARTESIAN_POINT ( 'NONE',  ( 28.77978050244509944, -3.315512618508630993, -7.939653947423660263 ) ) ;
#9873=CARTESIAN_POINT ( 'NONE',  ( 30.01874226414561875, -2.539271660970221944, -6.861505862736159145 ) ) ;
#9888=EDGE_LOOP ( 'NONE', ( #2288, #6255, #13536, #8728 ) ) ;
#9890=VECTOR ( 'NONE', #4936, 1000.000000000000000 ) ;
#9893=CARTESIAN_POINT ( 'NONE',  ( 32.85952466860454280, -1.897204703373130741, -7.033357778048658027 ) ) ;
#9898=CONICAL_SURFACE ( 'NONE', #12530, 3.425051884552432480, 0.7853981633974544962 ) ;
#9905=SURFACE_STYLE_USAGE ( .BOTH. , #15453 ) ;
#9916=CARTESIAN_POINT ( 'NONE',  ( 33.09223089549517738, -4.049888575955752579, -8.283357778048662468 ) ) ;
#9921=ORIENTED_EDGE ( 'NONE', *, *, #2539, .T. ) ;
#9930=FACE_OUTER_BOUND ( 'NONE', #16421, .T. ) ;
#9932=DIRECTION ( 'NONE',  ( -0.1196152422706618645, 0.9928203230275510771, 0.000000000000000000 ) ) ;
#9933=CARTESIAN_POINT ( 'NONE',  ( 33.73390066541284682, -2.518766455766908940, -3.283357778048662023 ) ) ;
#9934=CARTESIAN_POINT ( 'NONE',  ( 32.97402322492378346, -4.064130265842336165, -3.627061608673664672 ) ) ;
#9936=DIRECTION ( 'NONE',  ( -0.9928203230275510771, -0.1196152422706609902, -9.614813431917821547E-17 ) ) ;
#9938=CARTESIAN_POINT ( 'NONE',  ( 32.79901970863393501, -6.593096864778464017, -5.783357778048668685 ) ) ;
#9940=CARTESIAN_POINT ( 'NONE',  ( 26.62577407660990758, -3.575027854551694695, -3.627061608673662008 ) ) ;
#9943=ORIENTED_EDGE ( 'NONE', *, *, #408, .T. ) ;
#9951=CARTESIAN_POINT ( 'NONE',  ( 33.69269431359690969, -6.158264969628857166, -4.533357778048668685 ) ) ;
#9952=CARTESIAN_POINT ( 'NONE',  ( 31.45915434921569798, -2.992700983430681028, -7.939653947423660263 ) ) ;
#9955=DIRECTION ( 'NONE',  ( 0.6287809056569713118, 0.6925565483635240938, 0.3535533905932746745 ) ) ;
#9969=CARTESIAN_POINT ( 'NONE',  ( 27.55969062878875064, -7.234529412811931515, -5.783357778048668685 ) ) ;
#9974=EDGE_CURVE ( 'NONE', #3987, #13923, #590, .T. ) ;
#9977=ORIENTED_EDGE ( 'NONE', *, *, #16698, .F. ) ;
#9982=CARTESIAN_POINT ( 'NONE',  ( 31.24221605398236790, -5.726592414339752857, -8.283357778048662468 ) ) ;
#9984=CARTESIAN_POINT ( 'NONE',  ( 26.01652455409633902, -4.902371455920926380, -5.783357778048663356 ) ) ;
#9996=CARTESIAN_POINT ( 'NONE',  ( 30.60493568430522160, -6.867637522466304212, -5.113484796970860558 ) ) ;
#10000=DIRECTION ( 'NONE',  ( -0.1196152422706606572, 0.9928203230275512992, 0.000000000000000000 ) ) ;
#10004=CARTESIAN_POINT ( 'NONE',  ( 32.28234893270314387, -5.401404424200516807, -7.939653947423664704 ) ) ;
#10010=CARTESIAN_POINT ( 'NONE',  ( 27.30005507882132676, -4.747731375419166788, -3.627061608673664672 ) ) ;
#10013=CARTESIAN_POINT ( 'NONE',  ( 31.08763465596552322, -1.773323841400983758, -5.113484796970854340 ) ) ;
#10022=CARTESIAN_POINT ( 'NONE',  ( 26.83664947211162399, -6.984282976826746037, -4.533357778048668685 ) ) ;
#10027=CARTESIAN_POINT ( 'NONE',  ( 32.01513846370018967, -2.298745344637636912, -4.705209693361161349 ) ) ;
#10028=EDGE_CURVE ( 'NONE', #14403, #13578, #10803, .T. ) ;
#10029=CARTESIAN_POINT ( 'NONE',  ( 26.10492286888475633, -5.636087676172646610, -8.120510362352304057 ) ) ;
#10041=CARTESIAN_POINT ( 'NONE',  ( 33.46007730730551799, -5.886481946178435010, -4.705209693361169343 ) ) ;
#10042=CARTESIAN_POINT ( 'NONE',  ( 29.16815758536418102, -2.004582921727632971, -5.783357778048664244 ) ) ;
#10056=CARTESIAN_POINT ( 'NONE',  ( 25.95642634701329499, -4.403549397486667516, -3.686412874245489135 ) ) ;
#10058=DIRECTION ( 'NONE',  ( -0.1196152422706610735, 0.9928203230275511881, 0.000000000000000000 ) ) ;
#10070=CARTESIAN_POINT ( 'NONE',  ( 29.27960797773944179, -6.689954721521948144, -4.533357778048668685 ) ) ;
#10073=VECTOR ( 'NONE', #6993, 999.9999999999998863 ) ;
#10074=CARTESIAN_POINT ( 'NONE',  ( 32.26287188679368967, -2.695996373064596607, -8.283357778048658915 ) ) ;
#10086=CARTESIAN_POINT ( 'NONE',  ( 26.30108762358334928, -7.264277791658039440, -6.611981523323152032 ) ) ;
#10093=SHAPE_DEFINITION_REPRESENTATION ( #17552, #2651 ) ;
#10096=CARTESIAN_POINT ( 'NONE',  ( 32.82963640218302004, -5.962437625020304388, -4.705209693361169343 ) ) ;
#10103=CARTESIAN_POINT ( 'NONE',  ( 26.24062359194589078, -6.129313013101781671, -3.627061608673667781 ) ) ;
#10104=ORIENTED_EDGE ( 'NONE', *, *, #4806, .F. ) ;
#10115=CARTESIAN_POINT ( 'NONE',  ( 26.10855331130634127, -2.710563430764044490, -4.533357778048659803 ) ) ;
#10118=CARTESIAN_POINT ( 'NONE',  ( 31.25770402584614516, -1.763030703431812674, -5.783357778048658027 ) ) ;
#10121=CARTESIAN_POINT ( 'NONE',  ( 25.84832697747033592, -3.506312147857040706, -7.581167935121603918 ) ) ;
#10125=EDGE_LOOP ( 'NONE', ( #10126, #14543, #16749, #12783 ) ) ;
#10126=ORIENTED_EDGE ( 'NONE', *, *, #12099, .F. ) ;
#10136=CARTESIAN_POINT ( 'NONE',  ( 32.32618902979206865, -6.650063623909865385, -5.783357778048669573 ) ) ;
#10138=FACE_OUTER_BOUND ( 'NONE', #8768, .T. ) ;
#10140=PLANE ( 'NONE',  #1227 ) ;
#10151=CARTESIAN_POINT ( 'NONE',  ( 26.49461065740898391, -7.352653653197164907, -5.783357778048668685 ) ) ;
#10154=AXIS2_PLACEMENT_3D ( 'NONE', #4171, #8323, #9500 ) ;
#10157=CARTESIAN_POINT ( 'NONE',  ( 33.15485366002904755, -6.560422763297783177, -5.783357778048663356 ) ) ;
#10168=CARTESIAN_POINT ( 'NONE',  ( 29.34405387406022570, -7.019548880150045633, -5.113484796970862334 ) ) ;
#10171=ORIENTED_EDGE ( 'NONE', *, *, #13028, .T. ) ;
#10172=CARTESIAN_POINT ( 'NONE',  ( 30.58169613980036772, -2.898544849976259385, -3.283357778048662023 ) ) ;
#10180=EDGE_CURVE ( 'NONE', #7075, #3342, #1457, .T. ) ;
#10181=EDGE_LOOP ( 'NONE', ( #11392, #5979, #3930, #14896 ) ) ;
#10182=CARTESIAN_POINT ( 'NONE',  ( 25.41044654184514329, -5.982623484807521486, -5.783357778048664244 ) ) ;
#10188=EDGE_CURVE ( 'NONE', #3946, #3342, #7382, .T. ) ;
#10193=CARTESIAN_POINT ( 'NONE',  ( 32.80318959510331212, -2.203800746085299522, -4.705209693361160461 ) ) ;
#10202=CARTESIAN_POINT ( 'NONE',  ( 25.83772294520678159, -3.669972453104032084, -3.627061608673662896 ) ) ;
#10205=CARTESIAN_POINT ( 'NONE',  ( 31.97277696464621854, -6.702839660918840536, -5.783357778048663356 ) ) ;
#10209=CYLINDRICAL_SURFACE ( 'NONE', #11572, 2.500000000000001776 ) ;
#10212=CARTESIAN_POINT ( 'NONE',  ( 27.53837573810956130, -6.172832027328289506, -8.283357778048662468 ) ) ;
#10216=CARTESIAN_POINT ( 'NONE',  ( 29.60297508593253468, -5.724216059278466773, -7.939653947423664704 ) ) ;
#10217=CARTESIAN_POINT ( 'NONE',  ( 26.60838078660069428, -6.085005533777348319, -7.939653947423662927 ) ) ;
#10229=CARTESIAN_POINT ( 'NONE',  ( 26.49461065740898036, -7.352653653197164019, -5.783357778048668685 ) ) ;
#10257=CARTESIAN_POINT ( 'NONE',  ( 28.41265020943543362, -1.706058464416624787, -5.783357778048658027 ) ) ;
#10259=CARTESIAN_POINT ( 'NONE',  ( 31.89397184978405519, -6.712334120981523711, -5.783357778048663356 ) ) ;
#10262=ORIENTED_EDGE ( 'NONE', *, *, #17889, .T. ) ;
#10267=VERTEX_POINT ( 'NONE', #983 ) ;
#10272=CARTESIAN_POINT ( 'NONE',  ( 41.45058359766582612, -3.639327173243837255, -4.757684611182616763 ) ) ;
#10273=EDGE_CURVE ( 'NONE', #7301, #8853, #6144, .T. ) ;
#10278=CARTESIAN_POINT ( 'NONE',  ( 28.89355063163679915, -2.047864499088824175, -5.783357778048658027 ) ) ;
#10279=CARTESIAN_POINT ( 'NONE',  ( 38.64694918415791136, -1.054552983374778208, -9.283357778048653586 ) ) ;
#10284=CARTESIAN_POINT ( 'NONE',  ( 26.34117031759772942, -2.982346454214467535, -4.705209693361161349 ) ) ;
#10289=ORIENTED_EDGE ( 'NONE', *, *, #6823, .F. ) ;
#10295=CARTESIAN_POINT ( 'NONE',  ( 25.84216048658649001, -4.923378882637265974, -3.283357778048664688 ) ) ;
#10298=CARTESIAN_POINT ( 'NONE',  ( 28.36401332423200827, -6.500457016816879374, -6.861505862736166250 ) ) ;
#10302=ORIENTED_EDGE ( 'NONE', *, *, #8574, .T. ) ;
#10303=ORIENTED_EDGE ( 'NONE', *, *, #14347, .T. ) ;
#10304=EDGE_CURVE ( 'NONE', #12046, #4105, #16989, .T. ) ;
#10310=CARTESIAN_POINT ( 'NONE',  ( 31.55553118839817728, -4.235030543236534939, -7.939653947423662039 ) ) ;
#10316=CARTESIAN_POINT ( 'NONE',  ( 27.84978555093622177, -3.227686124957687586, -8.283357778048660691 ) ) ;
#10317=EDGE_LOOP ( 'NONE', ( #17218, #7152, #9834, #7474 ) ) ;
#10338=( BOUNDED_CURVE ( )  B_SPLINE_CURVE ( 2, ( #15629, #7297, #1951, #670, #7565, #15728, #13091, #3303, #6282 ),
 .UNSPECIFIED., .F., .F. ) 
 B_SPLINE_CURVE_WITH_KNOTS ( ( 3, 2, 2, 2, 3 ),
 ( 0.3269230769230769273, 0.3333333333333333148, 0.3461538461538461453, 0.3589743589743589758, 0.3653846153846154188 ),
 .UNSPECIFIED. ) 
 CURVE ( )  GEOMETRIC_REPRESENTATION_ITEM ( )  RATIONAL_B_SPLINE_CURVE ( ( 0.9330127018922194093, 0.9330127018922194093, 1.000000000000000000, 0.8660254037844387076, 1.000000000000000000, 0.8660254037844387076, 1.000000000000000000, 0.9330127018922190762, 0.9330127018922194093 ) ) 
 REPRESENTATION_ITEM ( '' )  );
#10345=CARTESIAN_POINT ( 'NONE',  ( 29.18195272205665347, -2.340279496617377664, -4.533357778048659803 ) ) ;
#10346=DIRECTION ( 'NONE',  ( 0.9928203230275512992, 0.1196152422706610180, 4.006172263299093133E-17 ) ) ;
#10362=DIRECTION ( 'NONE',  ( 0.9928203230275512992, 0.1196152422706610180, 4.006172263299093133E-17 ) ) ;
#10364=CARTESIAN_POINT ( 'NONE',  ( 30.81132015408399027, -5.578634341498224458, -3.627061608673668225 ) ) ;
#10375=ORIENTED_EDGE ( 'NONE', *, *, #13725, .F. ) ;
#10378=CARTESIAN_POINT ( 'NONE',  ( 27.16987539990068612, -2.245336462116964249, -6.453230759126464378 ) ) ;
#10379=VERTEX_POINT ( 'NONE', #17868 ) ;
#10386=EDGE_CURVE ( 'NONE', #17484, #16733, #8220, .T. ) ;
#10387=CARTESIAN_POINT ( 'NONE',  ( 30.76748005699505129, -4.329975141788874993, -7.939653947423662039 ) ) ;
#10391=CARTESIAN_POINT ( 'NONE',  ( 26.47269060886452507, -6.728324053342490174, -6.861505862736166250 ) ) ;
#10398=EDGE_LOOP ( 'NONE', ( #2770, #7593, #5353, #519 ) ) ;
#10408=CARTESIAN_POINT ( 'NONE',  ( 27.86926259684567597, -5.933094176093606897, -7.939653947423664704 ) ) ;
#10417=CARTESIAN_POINT ( 'NONE',  ( 31.41531425212677675, -1.744041783721344219, -5.783357778048658915 ) ) ;
#10422=CARTESIAN_POINT ( 'NONE',  ( 33.00219691583784964, -5.514549477365426888, -3.283357778048667797 ) ) ;
#10425=FACE_BOUND ( 'NONE', #14920, .T. ) ;
#10434=MECHANICAL_DESIGN_GEOMETRIC_PRESENTATION_REPRESENTATION('',(#15961),#15076);
#10436=CARTESIAN_POINT ( 'NONE',  ( 26.04653150877178902, -5.151432644682725659, -3.575219446611406227 ) ) ;
#10437=FACE_OUTER_BOUND ( 'NONE', #10802, .T. ) ;
#10439=CARTESIAN_POINT ( 'NONE',  ( 29.23078034989804763, -4.515117109069654688, -8.283357778048662468 ) ) ;
#10440=CARTESIAN_POINT ( 'NONE',  ( 31.25770402584614871, -1.763030703431812451, -5.783357778048658915 ) ) ;
#10442=EDGE_LOOP ( 'NONE', ( #7334, #195, #10699, #7519 ) ) ;
#10444=CARTESIAN_POINT ( 'NONE',  ( 26.78782184427022983, -4.809445364374452581, -8.283357778048662468 ) ) ;
#10450=CARTESIAN_POINT ( 'NONE',  ( 25.95642634701329499, -4.403549397486667516, -3.686412874245489135 ) ) ;
#10461=CARTESIAN_POINT ( 'NONE',  ( 29.67743187657054449, -6.342216019229654833, -4.705209693361169343 ) ) ;
#10467=CARTESIAN_POINT ( 'NONE',  ( 32.29220775574281532, -1.628196571319322050, -6.453230759126467042 ) ) ;
#10477=CARTESIAN_POINT ( 'NONE',  ( 31.53813789838894621, -6.745008222462202774, -5.783357778048668685 ) ) ;
#10479=CIRCLE ( 'NONE', #8176, 2.499999999999999556 ) ;
#10481=CARTESIAN_POINT ( 'NONE',  ( 28.25893984004492765, -6.513116296623863377, -4.705209693361168455 ) ) ;
#10486=DIRECTION ( 'NONE',  ( -0.4714752725849062909, -0.8818792816145463176, -1.010345934383541768E-15 ) ) ;
#10487=VECTOR ( 'NONE', #15737, 1000.000000000000114 ) ;
#10490=VECTOR ( 'NONE', #15888, 1000.000000000000114 ) ;
#10499=CARTESIAN_POINT ( 'NONE',  ( 30.28142597461332741, -2.507623461452779701, -4.705209693361160461 ) ) ;
#10500=CARTESIAN_POINT ( 'NONE',  ( 30.33776104811456165, -2.201027418740610919, -7.033357778048658027 ) ) ;
#10509=CARTESIAN_POINT ( 'NONE',  ( 32.80318959510331212, -2.203800746085299522, -4.705209693361160461 ) ) ;
#10511=CARTESIAN_POINT ( 'NONE',  ( 38.70301816123731697, -5.700001250565214228, -1.783357778048662690 ) ) ;
#10513=EDGE_CURVE ( 'NONE', #15016, #13726, #5521, .T. ) ;
#10520=CARTESIAN_POINT ( 'NONE',  ( 28.71361296893772774, -7.095504558991913235, -5.113484796970856117 ) ) ;
#10529=CARTESIAN_POINT ( 'NONE',  ( 28.75424055680402802, -6.753251120556833520, -7.033357778048666908 ) ) ;
#10530=CARTESIAN_POINT ( 'NONE',  ( 33.27602027394517847, -2.146833986953896822, -4.705209693361161349 ) ) ;
#10540=EDGE_CURVE ( 'NONE', #9716, #757, #2927, .T. ) ;
#10546=CARTESIAN_POINT ( 'NONE',  ( 29.76058531221316628, -5.705227139567997874, -7.939653947423664704 ) ) ;
#10552=EDGE_CURVE ( 'NONE', #3859, #1701, #11967, .T. ) ;
#10560=CARTESIAN_POINT ( 'NONE',  ( 28.19013153391124860, -7.158573733970061248, -5.783357778048657138 ) ) ;
#10562=CARTESIAN_POINT ( 'NONE',  ( 32.65880277236253448, -4.102108105263264193, -7.939653947423662039 ) ) ;
#10566=CARTESIAN_POINT ( 'NONE',  ( 28.75786045390062995, -2.691183018653962034, -6.861505862736159145 ) ) ;
#10579=CARTESIAN_POINT ( 'NONE',  ( 28.93739072872572393, -3.296523698798161650, -7.939653947423660263 ) ) ;
#10581=CARTESIAN_POINT ( 'NONE',  ( 33.18226487515251222, -2.585227674546096033, -3.283357778048662023 ) ) ;
#10587=CARTESIAN_POINT ( 'NONE',  ( 31.66930131758986633, -2.967382423816733894, -3.627061608673662008 ) ) ;
#10592=CARTESIAN_POINT ( 'NONE',  ( 32.41296236253129592, -1.951006642345344044, -4.533357778048659803 ) ) ;
#10609=CARTESIAN_POINT ( 'NONE',  ( 29.74110826630370497, -2.999819088432076786, -8.283357778048658915 ) ) ;
#10610=CARTESIAN_POINT ( 'NONE',  ( 30.86385689617753059, -5.572304701594727128, -7.939653947423662927 ) ) ;
#10613=CARTESIAN_POINT ( 'NONE',  ( 38.70301816123731697, -5.700001250565210675, -9.783357778048662468 ) ) ;
#10624=CARTESIAN_POINT ( 'NONE',  ( 30.91186687973582536, -2.431667782610909434, -4.705209693361160461 ) ) ;
#10626=CARTESIAN_POINT ( 'NONE',  ( 33.30246708102489350, -5.905470865888903020, -4.705209693361168455 ) ) ;
#10630=EDGE_LOOP ( 'NONE', ( #11292, #8722, #10303, #6470 ) ) ;
#10634=ORIENTED_EDGE ( 'NONE', *, *, #1946, .T. ) ;
#10635=CARTESIAN_POINT ( 'NONE',  ( 33.16732689266149237, -6.221561368663743430, -7.033357778048666908 ) ) ;
#10636=AXIS2_PLACEMENT_3D ( 'NONE', #17166, #4889, #11872 ) ;
#10641=VECTOR ( 'NONE', #3746, 1000.000000000000114 ) ;
#10648=DIRECTION ( 'NONE',  ( -0.1196152422706610735, 0.9928203230275511881, 0.000000000000000000 ) ) ;
#10650=CARTESIAN_POINT ( 'NONE',  ( 32.26971135134834867, -1.630906943779925955, -5.113484796970855228 ) ) ;
#10652=VERTEX_POINT ( 'NONE', #9582 ) ;
#10660=CARTESIAN_POINT ( 'NONE',  ( 28.49970350196817392, -5.857138497251738407, -7.939653947423664704 ) ) ;
#10663=DIRECTION ( 'NONE',  ( 0.9928203230275510771, 0.1196152422706609902, 4.006172263299092517E-17 ) ) ;
#10669=CARTESIAN_POINT ( 'NONE',  ( 30.60986983071443390, -4.348964061499348333, -3.627061608673664672 ) ) ;
#10670=EDGE_LOOP ( 'NONE', ( #4779, #652, #5462, #4566 ) ) ;
#10689=CARTESIAN_POINT ( 'NONE',  ( 25.95846283556873502, -3.455553161483296609, -8.283357778048658915 ) ) ;
#10692=CARTESIAN_POINT ( 'NONE',  ( 33.17547354829333983, -5.293800545841212291, -3.627061608673667781 ) ) ;
#10694=ADVANCED_FACE ( 'NONE', ( #5506 ), #34, .T. ) ;
#10699=ORIENTED_EDGE ( 'NONE', *, *, #4091, .T. ) ;
#10712=CARTESIAN_POINT ( 'NONE',  ( 26.62577407660990758, -3.575027854551694695, -3.627061608673662008 ) ) ;
#10714=CARTESIAN_POINT ( 'NONE',  ( 25.93714794488954212, -2.393855775999666591, -5.783357778048658027 ) ) ;
#10718=ORIENTED_EDGE ( 'NONE', *, *, #8787, .T. ) ;
#10725=EDGE_CURVE ( 'NONE', #13835, #2767, #10860, .T. ) ;
#10740=EDGE_LOOP ( 'NONE', ( #2824, #11549, #119, #8488 ) ) ;
#10748=CARTESIAN_POINT ( 'NONE',  ( 29.14000323013032556, -2.007974965528672495, -6.453230759126468818 ) ) ;
#10751=CARTESIAN_POINT ( 'NONE',  ( 29.02054416436834217, -2.659534819136519790, -4.705209693361160461 ) ) ;
#10753=CARTESIAN_POINT ( 'NONE',  ( 32.51061761821408425, -6.300681867249914525, -4.533357778048668685 ) ) ;
#10760=ADVANCED_FACE ( 'NONE', ( #12804, #14447 ), #11430, .T. ) ;
#10761=CARTESIAN_POINT ( 'NONE',  ( 29.54591158530375239, -2.596238420101622868, -6.861505862736158257 ) ) ;
#10770=LINE ( 'NONE', #3991, #16829 ) ;
#10782=CARTESIAN_POINT ( 'NONE',  ( 26.61898274975073164, -6.283600725846810953, -3.283357778048667797 ) ) ;
#10783=CARTESIAN_POINT ( 'NONE',  ( 33.40754056521197413, -5.892811586081919906, -6.861505862736166250 ) ) ;
#10787=DIRECTION ( 'NONE',  ( 0.1196152422706609625, -0.9928203230275510771, 0.000000000000000000 ) ) ;
#10794=ORIENTED_EDGE ( 'NONE', *, *, #11581, .F. ) ;
#10799=CARTESIAN_POINT ( 'NONE',  ( 26.37178701114681800, -2.351687214456304353, -5.783357778048658027 ) ) ;
#10802=EDGE_LOOP ( 'NONE', ( #9943, #2585, #7250, #4088 ) ) ;
#10803=( BOUNDED_CURVE ( )  B_SPLINE_CURVE ( 2, ( #645, #8614, #5796, #14427, #551, #4621, #12966, #14146, #6068 ),
 .UNSPECIFIED., .F., .T. ) 
 B_SPLINE_CURVE_WITH_KNOTS ( ( 3, 2, 2, 2, 3 ),
 ( 0.2884615384615384914, 0.2948717948717948789, 0.3076923076923077094, 0.3205128205128205399, 0.3269230769230769273 ),
 .UNSPECIFIED. ) 
 CURVE ( )  GEOMETRIC_REPRESENTATION_ITEM ( )  RATIONAL_B_SPLINE_CURVE ( ( 0.9330127018922194093, 0.9330127018922196314, 1.000000000000000000, 0.8660254037844387076, 1.000000000000000000, 0.8660254037844387076, 1.000000000000000000, 0.9330127018922194093, 0.9330127018922194093 ) ) 
 REPRESENTATION_ITEM ( '' )  );
#10804=APPLICATION_CONTEXT ( 'automotive_design' ) ;
#10811=CARTESIAN_POINT ( 'NONE',  ( 38.15053902264412500, -1.114360604510109098, -1.783357778048662912 ) ) ;
#10834=CARTESIAN_POINT ( 'NONE',  ( 26.01652455409633902, -4.902371455920926380, -5.783357778048663356 ) ) ;
#10849=CARTESIAN_POINT ( 'NONE',  ( 29.02054416436834217, -2.659534819136519790, -4.705209693361160461 ) ) ;
#10857=CARTESIAN_POINT ( 'NONE',  ( 41.90164972253716513, -2.988527579590351646, -5.783357778048662468 ) ) ;
#10860=B_SPLINE_CURVE_WITH_KNOTS ( 'NONE', 1,
 ( #5327, #1276 ),
 .UNSPECIFIED., .F., .F.,
 ( 2, 2 ),
 ( 0.000000000000000000, 1.000000000000000000 ),
 .UNSPECIFIED. ) ;
#10867=FACE_OUTER_BOUND ( 'NONE', #13983, .T. ) ;
#10868=CARTESIAN_POINT ( 'NONE',  ( 26.07857582428556853, -4.894895503279006022, -8.283357778048662468 ) ) ;
#10869=CARTESIAN_POINT ( 'NONE',  ( 28.38593337277646711, -7.124786616671554107, -5.783357778048668685 ) ) ;
#10871=LINE ( 'NONE', #8000, #17545 ) ;
#10877=ORIENTED_EDGE ( 'NONE', *, *, #13165, .F. ) ;
#10885=CARTESIAN_POINT ( 'NONE',  ( 26.19678349485696955, -4.880653813392439311, -3.627061608673664672 ) ) ;
#10894=DIRECTION ( 'NONE',  ( -0.9928203230275511881, -0.1196152422706606572, -1.761484381769779444E-15 ) ) ;
#10913=CARTESIAN_POINT ( 'NONE',  ( 28.79925754835455010, -6.020920669644549861, -8.283357778048664244 ) ) ;
#10921=CARTESIAN_POINT ( 'NONE',  ( 25.98779870451785001, -2.387753359738024272, -6.453230759126469707 ) ) ;
#10923=CARTESIAN_POINT ( 'NONE',  ( 29.84999239022537409, -5.894327871574777333, -3.283357778048667797 ) ) ;
#10930=CARTESIAN_POINT ( 'NONE',  ( 27.12922144900085186, -2.887401855662130146, -4.705209693361160461 ) ) ;
#10943=CARTESIAN_POINT ( 'NONE',  ( 37.87429945334753256, 1.178459718517443022, -5.783357778048661579 ) ) ;
#10944=CARTESIAN_POINT ( 'NONE',  ( 28.98992747081925359, -3.290194058894681639, -3.627061608673662896 ) ) ;
#10948=DIRECTION ( 'NONE',  ( 0.9928203230275512992, 0.1196152422706610180, 4.006172263299093133E-17 ) ) ;
#10959=CARTESIAN_POINT ( 'NONE',  ( 28.87615734162756453, -4.557842178314484016, -7.939653947423662039 ) ) ;
#10962=( BOUNDED_CURVE ( )  B_SPLINE_CURVE ( 2, ( #14238, #373, #17059, #6982, #8521, #7174, #274, #5787, #10042 ),
 .UNSPECIFIED., .F., .T. ) 
 B_SPLINE_CURVE_WITH_KNOTS ( ( 3, 2, 2, 2, 3 ),
 ( 0.4423076923076923461, 0.4487179487179487336, 0.4615384615384615641, 0.4743589743589743390, 0.4807692307692307820 ),
 .UNSPECIFIED. ) 
 CURVE ( )  GEOMETRIC_REPRESENTATION_ITEM ( )  RATIONAL_B_SPLINE_CURVE ( ( 0.9330127018922194093, 0.9330127018922196314, 1.000000000000000000, 0.8660254037844387076, 1.000000000000000000, 0.8660254037844387076, 1.000000000000000000, 0.9330127018922190762, 0.9330127018922194093 ) ) 
 REPRESENTATION_ITEM ( '' )  );
#10975=CARTESIAN_POINT ( 'NONE',  ( 27.04606801335823718, -3.524390735323772006, -7.939653947423660263 ) ) ;
#10977=EDGE_CURVE ( 'NONE', #7401, #15874, #4618, .T. ) ;
#10985=CARTESIAN_POINT ( 'NONE',  ( 27.42949161418789217, -3.278323244185609830, -3.283357778048662023 ) ) ;
#10994=CARTESIAN_POINT ( 'NONE',  ( 28.79241808379989465, -7.086010098929231837, -5.113484796970862334 ) ) ;
#11017=CARTESIAN_POINT ( 'NONE',  ( 29.62480591732145996, -4.467644809586046151, -3.283357778048664688 ) ) ;
#11019=CARTESIAN_POINT ( 'NONE',  ( 25.71748644841968456, -2.420320648352046078, -5.783357778048663356 ) ) ;
#11025=CARTESIAN_POINT ( 'NONE',  ( 28.30694982360322953, -3.372479377640031473, -7.939653947423660263 ) ) ;
#11036=CARTESIAN_POINT ( 'NONE',  ( 27.49697864365563760, -2.843094376337701679, -6.861505862736159145 ) ) ;
#11041=CARTESIAN_POINT ( 'NONE',  ( 25.71748644841968456, -2.420320648352046078, -5.783357778048663356 ) ) ;
#11043=EDGE_LOOP ( 'NONE', ( #7050, #4967, #4196, #1967 ) ) ;
#11052=CARTESIAN_POINT ( 'NONE',  ( 30.13703915187255689, -4.405930820630744371, -7.939653947423662039 ) ) ;
#11064=CIRCLE ( 'NONE', #2694, 2.500000000000001776 ) ;
#11068=CARTESIAN_POINT ( 'NONE',  ( 27.00222791626931595, -2.275731535614434531, -5.783357778048658027 ) ) ;
#11072=EDGE_CURVE ( 'NONE', #5290, #16997, #13530, .T. ) ;
#11079=CARTESIAN_POINT ( 'NONE',  ( 26.31176419598820360, -7.352894575460818594, -6.182016197336221985 ) ) ;
#11083=CARTESIAN_POINT ( 'NONE',  ( 28.58911057998038885, -6.046239229258517867, -3.283357778048667797 ) ) ;
#11100=FACE_OUTER_BOUND ( 'NONE', #7515, .T. ) ;
#11101=CARTESIAN_POINT ( 'NONE',  ( 26.63030083514515312, -6.709335133632020387, -6.861505862736167138 ) ) ;
#11103=CARTESIAN_POINT ( 'NONE',  ( 28.79925754835455010, -6.020920669644549861, -8.283357778048662468 ) ) ;
#11107=CARTESIAN_POINT ( 'NONE',  ( 29.38830135902312080, -2.615227339812091767, -6.861505862736159145 ) ) ;
#11108=CARTESIAN_POINT ( 'NONE',  ( 28.41655006632555569, -6.494127376913395366, -4.705209693361169343 ) ) ;
#11113=ORIENTED_EDGE ( 'NONE', *, *, #501, .F. ) ;
#11119=CARTESIAN_POINT ( 'NONE',  ( 30.12381574833269937, -2.526612381163247267, -4.705209693361161349 ) ) ;
#11122=LINE ( 'NONE', #5693, #13639 ) ;
#11130=CARTESIAN_POINT ( 'NONE',  ( 31.26353094466156080, -6.788289799823394866, -5.783357778048663356 ) ) ;
#11132=CARTESIAN_POINT ( 'NONE',  ( 28.73594040535617467, -2.066853418799292630, -5.783357778048658915 ) ) ;
#11146=DIRECTION ( 'NONE',  ( -0.9985081203071058953, 0.05460342187784718998, -9.468742811518590322E-17 ) ) ;
#11148=CARTESIAN_POINT ( 'NONE',  ( 30.33776104811456165, -2.201027418740610919, -7.033357778048658027 ) ) ;
#11183=CARTESIAN_POINT ( 'NONE',  ( 27.65911562847151117, -5.958412735707574015, -3.627061608673668225 ) ) ;
#11185=CARTESIAN_POINT ( 'NONE',  ( 30.45035428628836627, -2.914368949527523789, -8.283357778048658915 ) ) ;
#11187=EDGE_CURVE ( 'NONE', #6885, #15376, #8435, .T. ) ;
#11191=CARTESIAN_POINT ( 'NONE',  ( 32.75517961154501023, -5.344437665069116328, -7.939653947423664704 ) ) ;
#11205=CARTESIAN_POINT ( 'NONE',  ( 29.62489513447700062, -6.348545659133139729, -6.861505862736166250 ) ) ;
#11218=FACE_OUTER_BOUND ( 'NONE', #8264, .T. ) ;
#11220=CARTESIAN_POINT ( 'NONE',  ( 29.82181869931131146, -4.443908660051686610, -3.627061608673664672 ) ) ;
#11221=EDGE_LOOP ( 'NONE', ( #6702, #15971, #2759, #6746 ) ) ;
#11223=FACE_OUTER_BOUND ( 'NONE', #10398, .T. ) ;
#11232=EDGE_CURVE ( 'NONE', #17258, #9429, #13951, .T. ) ;
#11238=CARTESIAN_POINT ( 'NONE',  ( 32.29295089585319545, -5.599999616269980329, -3.283357778048667797 ) ) ;
#11240=CARTESIAN_POINT ( 'NONE',  ( 31.59864285835955400, -2.049116061056871274, -7.033357778048658027 ) ) ;
#11258=CARTESIAN_POINT ( 'NONE',  ( 33.13163345120441505, -4.045141346131868154, -3.627061608673664672 ) ) ;
#11263=AXIS2_PLACEMENT_3D ( 'NONE', #5760, #12933, #347 ) ;
#11264=EDGE_LOOP ( 'NONE', ( #7962, #12582, #9547, #9145 ) ) ;
#11273=( BOUNDED_CURVE ( )  B_SPLINE_CURVE ( 2, ( #2783, #13581, #13755, #15021, #12307, #10913, #1163, #16659, #6682 ),
 .UNSPECIFIED., .F., .T. ) 
 B_SPLINE_CURVE_WITH_KNOTS ( ( 3, 2, 2, 2, 3 ),
 ( 0.5576923076923077094, 0.5641025641025640969, 0.5769230769230768718, 0.5897435897435897578, 0.5961538461538461453 ),
 .UNSPECIFIED. ) 
 CURVE ( )  GEOMETRIC_REPRESENTATION_ITEM ( )  RATIONAL_B_SPLINE_CURVE ( ( 0.9330127018922194093, 0.9330127018922194093, 1.000000000000000000, 0.8660254037844387076, 1.000000000000000000, 0.8660254037844387076, 1.000000000000000000, 0.9330127018922194093, 0.9330127018922194093 ) ) 
 REPRESENTATION_ITEM ( '' )  );
#11277=CARTESIAN_POINT ( 'NONE',  ( 30.63309003953906995, -6.864245478665264244, -5.783357778048663356 ) ) ;
#11280=CARTESIAN_POINT ( 'NONE',  ( 30.75815651034531584, -7.238725614818142695, -5.783357778048669573 ) ) ;
#11281=COLOUR_RGB ( '', 0.31764706, 0.68627451, 0.89019608) ;
#11285=CARTESIAN_POINT ( 'NONE',  ( 32.64557936882268052, -2.222789665795767089, -4.705209693361161349 ) ) ;
#11287=CARTESIAN_POINT ( 'NONE',  ( 26.49878054387835746, -2.963357534503999968, -4.705209693361160461 ) ) ;
#11289=CARTESIAN_POINT ( 'NONE',  ( 27.48088551392658729, -7.244023872874614689, -5.783357778048657138 ) ) ;
#11292=ORIENTED_EDGE ( 'NONE', *, *, #9234, .F. ) ;
#11299=CARTESIAN_POINT ( 'NONE',  ( 28.99436501219896201, -4.543600488427916417, -3.283357778048664688 ) ) ;
#11300=CARTESIAN_POINT ( 'NONE',  ( 32.07220196432897552, -5.426722983814484813, -3.627061608673668225 ) ) ;
#11306=EDGE_CURVE ( 'NONE', #6149, #10652, #17705, .T. ) ;
#11316=CARTESIAN_POINT ( 'NONE',  ( 26.87106449706838873, -6.053357334259913181, -3.627061608673667781 ) ) ;
#11328=ORIENTED_EDGE ( 'NONE', *, *, #408, .F. ) ;
#11337=CARTESIAN_POINT ( 'NONE',  ( 31.43732351782677625, -4.249272233123119413, -3.283357778048664688 ) ) ;
#11342=VECTOR ( 'NONE', #11739, 1000.000000000000000 ) ;
#11362=CARTESIAN_POINT ( 'NONE',  ( 33.56515079149260572, -5.873822666371450119, -6.861505862736167138 ) ) ;
#11363=CARTESIAN_POINT ( 'NONE',  ( 41.54280399572520821, -0.01006661050770166557, -5.783357778048662468 ) ) ;
#11370=EDGE_LOOP ( 'NONE', ( #989, #5631, #14204, #5396, #9673 ) ) ;
#11373=CARTESIAN_POINT ( 'NONE',  ( 42.32364987186199556, -2.937684895442014277, -5.783357778048662468 ) ) ;
#11383=CARTESIAN_POINT ( 'NONE',  ( 26.66770885555339987, -3.370103022578743612, -8.283357778048658915 ) ) ;
#11387=CARTESIAN_POINT ( 'NONE',  ( 32.56242593318007295, -2.859778545457410281, -7.939653947423660263 ) ) ;
#11388=VERTEX_POINT ( 'NONE', #9034 ) ;
#11390=CARTESIAN_POINT ( 'NONE',  ( 25.94629020164262556, -4.319418220471658465, -8.066408332899133171 ) ) ;
#11391=CARTESIAN_POINT ( 'NONE',  ( 26.66018910156667232, -2.644102211984857842, -4.533357778048659803 ) ) ;
#11392=ORIENTED_EDGE ( 'NONE', *, *, #9449, .F. ) ;
#11394=ORIENTED_EDGE ( 'NONE', *, *, #10513, .T. ) ;
#11399=CARTESIAN_POINT ( 'NONE',  ( 30.35023428074701002, -1.862166024106576057, -5.783357778048664244 ) ) ;
#11402=CARTESIAN_POINT ( 'NONE',  ( 32.90015225647083952, -1.554951264938056132, -5.113484796970854340 ) ) ;
#11403=CARTESIAN_POINT ( 'NONE',  ( 31.67382807612511542, -6.101689702897060030, -6.861505862736167138 ) ) ;
#11415=CARTESIAN_POINT ( 'NONE',  ( 26.25801688195511474, -3.619335333876111171, -7.939653947423660263 ) ) ;
#11430=PLANE ( 'NONE',  #12190 ) ;
#11434=CARTESIAN_POINT ( 'NONE',  ( 31.87265695910486230, -5.650636735497883478, -8.283357778048662468 ) ) ;
#11435=CARTESIAN_POINT ( 'NONE',  ( 29.08935247050201767, -2.014077381790315702, -5.783357778048658027 ) ) ;
#11445=ORIENTED_EDGE ( 'NONE', *, *, #7640, .F. ) ;
#11449=DIRECTION ( 'NONE',  ( -0.1196152422706610735, 0.9928203230275511881, 0.000000000000000000 ) ) ;
#11454=CARTESIAN_POINT ( 'NONE',  ( 33.32855701603872234, -2.140504347050403045, -6.861505862736158257 ) ) ;
#11461=CARTESIAN_POINT ( 'NONE',  ( 26.46816385032927599, -3.594016774262162706, -3.627061608673662896 ) ) ;
#11465=FACE_OUTER_BOUND ( 'NONE', #13816, .T. ) ;
#11471=CARTESIAN_POINT ( 'NONE',  ( 33.30246708102489350, -5.905470865888903020, -4.705209693361168455 ) ) ;
#11474=CARTESIAN_POINT ( 'NONE',  ( 32.04158527077989760, -6.057382223572642665, -4.705209693361168455 ) ) ;
#11476=EDGE_CURVE ( 'NONE', #5903, #317, #5288, .T. ) ;
#11481=CARTESIAN_POINT ( 'NONE',  ( 29.34898802046944155, -4.500875419183088866, -3.627061608673664672 ) ) ;
#11489=CARTESIAN_POINT ( 'NONE',  ( 31.24031073583692475, -4.273008382657478954, -3.627061608673664672 ) ) ;
#11491=CYLINDRICAL_SURFACE ( 'NONE', #5808, 2.500000000000001776 ) ;
#11492=CARTESIAN_POINT ( 'NONE',  ( 29.71979337562451207, -1.938121702948446323, -5.783357778048664244 ) ) ;
#11500=( BOUNDED_CURVE ( )  B_SPLINE_CURVE ( 2, ( #13164, #9086, #15797, #7723, #6359, #7823, #13446, #13354, #17740 ),
 .UNSPECIFIED., .F., .T. ) 
 B_SPLINE_CURVE_WITH_KNOTS ( ( 3, 2, 2, 2, 3 ),
 ( 0.01923076923076924918, 0.02564102564102564014, 0.03846153846153846367, 0.05128205128205128027, 0.05769230769230770939 ),
 .UNSPECIFIED. ) 
 CURVE ( )  GEOMETRIC_REPRESENTATION_ITEM ( )  RATIONAL_B_SPLINE_CURVE ( ( 0.9330127018922194093, 0.9330127018922195203, 1.000000000000000000, 0.8660254037844387076, 1.000000000000000000, 0.8660254037844387076, 1.000000000000000000, 0.9330127018922190762, 0.9330127018922194093 ) ) 
 REPRESENTATION_ITEM ( '' )  );
#11503=CARTESIAN_POINT ( 'NONE',  ( 27.12505156253147831, -7.276697974355292864, -5.783357778048668685 ) ) ;
#11504=EDGE_CURVE ( 'NONE', #16771, #4820, #4068, .T. ) ;
#11519=CARTESIAN_POINT ( 'NONE',  ( 28.91555989733679866, -4.553094948490599592, -3.283357778048664688 ) ) ;
#11523=CARTESIAN_POINT ( 'NONE',  ( 30.67935139548315604, -7.248220074880824981, -5.783357778048669573 ) ) ;
#11525=CARTESIAN_POINT ( 'NONE',  ( 31.92212620501791775, -6.708942077180482855, -6.453230759126470595 ) ) ;
#11529=DIRECTION ( 'NONE',  ( -0.1196152422706610735, 0.9928203230275511881, 0.000000000000000000 ) ) ;
#11532=ORIENTED_EDGE ( 'NONE', *, *, #8603, .T. ) ;
#11534=ORIENTED_EDGE ( 'NONE', *, *, #8787, .F. ) ;
#11538=CYLINDRICAL_SURFACE ( 'NONE', #2676, 2.500000000000001776 ) ;
#11540=CARTESIAN_POINT ( 'NONE',  ( 46.74613609540429593, -1.397631045209497103, -5.783357778048662468 ) ) ;
#11543=CARTESIAN_POINT ( 'NONE',  ( 26.64639396487419987, -2.308405637095112706, -5.783357778048658027 ) ) ;
#11549=ORIENTED_EDGE ( 'NONE', *, *, #1129, .T. ) ;
#11553=CARTESIAN_POINT ( 'NONE',  ( 38.43976950718546703, 0.6650622588958786663, -5.783357778048660691 ) ) ;
#11558=DIRECTION ( 'NONE',  ( -0.1196152422706599494, 0.9928203230275514102, 0.000000000000000000 ) ) ;
#11565=AXIS2_PLACEMENT_3D ( 'NONE', #3219, #4486, #10000 ) ;
#11567=CARTESIAN_POINT ( 'NONE',  ( 25.37303892199676270, -2.799178389412888546, -7.033357778048658027 ) ) ;
#11571=CARTESIAN_POINT ( 'NONE',  ( 28.24571643650507369, -4.633797857156355171, -7.939653947423662039 ) ) ;
#11572=AXIS2_PLACEMENT_3D ( 'NONE', #15756, #15387, #2974 ) ;
#11581=EDGE_CURVE ( 'NONE', #13923, #4502, #5838, .T. ) ;
#11585=CARTESIAN_POINT ( 'NONE',  ( 32.19919549706052209, -6.038393303862174655, -4.705209693361169343 ) ) ;
#11586=CARTESIAN_POINT ( 'NONE',  ( 30.35023428074701002, -1.862166024106576057, -5.783357778048664244 ) ) ;
#11605=CARTESIAN_POINT ( 'NONE',  ( 32.32036211097666012, -1.624804527518282748, -5.783357778048663356 ) ) ;
#11616=EDGE_CURVE ( 'NONE', #13615, #16315, #5725, .T. ) ;
#11622=CARTESIAN_POINT ( 'NONE',  ( 29.32081432955537892, -3.050456207659999475, -3.283357778048662023 ) ) ;
#11643=DIRECTION ( 'NONE',  ( 0.9928203230275511881, 0.1196152422706610180, 9.614813431917825245E-17 ) ) ;
#11644=CARTESIAN_POINT ( 'NONE',  ( 33.30663696749426350, -1.516174747195733863, -5.783357778048658027 ) ) ;
#11650=MECHANICAL_DESIGN_GEOMETRIC_PRESENTATION_REPRESENTATION('',(#17506),#13415);
#11652=CARTESIAN_POINT ( 'NONE',  ( 27.09860475545177039, -3.518061095420291995, -3.627061608673662896 ) ) ;
#11664=CARTESIAN_POINT ( 'NONE',  ( 25.96969170380761582, -2.000386719721422235, -5.783357778048658027 ) ) ;
#11668=CARTESIAN_POINT ( 'NONE',  ( 27.49697864365563760, -2.843094376337701679, -6.861505862736159145 ) ) ;
#11671=CARTESIAN_POINT ( 'NONE',  ( 32.47301885516785092, -2.670677813450649918, -3.283357778048662023 ) ) ;
#11681=CARTESIAN_POINT ( 'NONE',  ( 32.17274868998081416, -2.279756424927169345, -4.705209693361160461 ) ) ;
#11704=CARTESIAN_POINT ( 'NONE',  ( 29.69163902039066372, -1.941513746749485847, -6.453230759126468818 ) ) ;
#11709=CARTESIAN_POINT ( 'NONE',  ( 27.84978555093622177, -3.227686124957687586, -8.283357778048658915 ) ) ;
#11721=CARTESIAN_POINT ( 'NONE',  ( 25.83973938098743517, -3.435034105423886874, -4.207126410816434792 ) ) ;
#11728=CARTESIAN_POINT ( 'NONE',  ( 30.78487334700428590, -1.819997462563214263, -5.783357778048658027 ) ) ;
#11735=CARTESIAN_POINT ( 'NONE',  ( 25.58373587974369201, -2.446631813008643075, -5.783357778048658027 ) ) ;
#11739=DIRECTION ( 'NONE',  ( 0.6174492339697391641, 0.7866107318554600436, 0.000000000000000000 ) ) ;
#11741=ORIENTED_EDGE ( 'NONE', *, *, #419, .T. ) ;
#11748=CARTESIAN_POINT ( 'NONE',  ( 26.73899421642883567, -2.634607751922174224, -4.533357778048659803 ) ) ;
#11750=CARTESIAN_POINT ( 'NONE',  ( 39.47566789204768867, -7.933013952457433682, -5.783357778048662468 ) ) ;
#11752=CARTESIAN_POINT ( 'NONE',  ( 28.76238721243587193, -5.825490297734302381, -3.627061608673667781 ) ) ;
#11765=EDGE_CURVE ( 'NONE', #7873, #9123, #6553, .T. ) ;
#11767=CARTESIAN_POINT ( 'NONE',  ( 27.65458886993626564, -2.824105456627233224, -6.861505862736158257 ) ) ;
#11772=CARTESIAN_POINT ( 'NONE',  ( 27.53153627355490229, -7.237921456612971483, -5.113484796970862334 ) ) ;
#11777=CARTESIAN_POINT ( 'NONE',  ( 32.72003615946069743, -2.840789625746940938, -7.939653947423660263 ) ) ;
#11788=CARTESIAN_POINT ( 'NONE',  ( 28.05993251931039012, -3.202367565343740452, -3.283357778048662023 ) ) ;
#11789=EDGE_LOOP ( 'NONE', ( #14862, #13114, #7330, #12993 ) ) ;
#11791=CARTESIAN_POINT ( 'NONE',  ( 30.03080348965042745, -6.936809113706096319, -6.453230759126468818 ) ) ;
#11799=CARTESIAN_POINT ( 'NONE',  ( 26.58890374069123652, -3.379597482641427231, -8.283357778048658915 ) ) ;
#11800=CARTESIAN_POINT ( 'NONE',  ( 31.51621784984448738, -6.120678622607529817, -6.861505862736166250 ) ) ;
#11802=ORIENTED_EDGE ( 'NONE', *, *, #8574, .F. ) ;
#11809=CARTESIAN_POINT ( 'NONE',  ( 31.00882954110335632, -1.782818301463667598, -5.113484796970851676 ) ) ;
#11810=CARTESIAN_POINT ( 'NONE',  ( 25.75741033704265703, -2.751693534003876174, -5.973512092880350011 ) ) ;
#11820=CARTESIAN_POINT ( 'NONE',  ( 29.15206445563513071, -6.405512418264540209, -6.861505862736167138 ) ) ;
#11839=CARTESIAN_POINT ( 'NONE',  ( 31.41114436565740320, -6.133337902414513820, -4.705209693361168455 ) ) ;
#11843=CARTESIAN_POINT ( 'NONE',  ( 29.64681518302145591, -6.972875258987813574, -5.783357778048668685 ) ) ;
#11857=CARTESIAN_POINT ( 'NONE',  ( 25.17121605730381972, -3.996982838752419553, -5.783357778048664244 ) ) ;
#11860=CARTESIAN_POINT ( 'NONE',  ( 30.15443244188179150, -1.895953141405084086, -5.783357778048658027 ) ) ;
#11864=CARTESIAN_POINT ( 'NONE',  ( 32.37175601071535880, -5.590505156207296267, -3.283357778048667797 ) ) ;
#11869=CARTESIAN_POINT ( 'NONE',  ( 33.56515079149260572, -5.873822666371450119, -6.861505862736167138 ) ) ;
#11872=DIRECTION ( 'NONE',  ( -0.1196152422706610735, 0.9928203230275511881, 0.000000000000000000 ) ) ;
#11892=CARTESIAN_POINT ( 'NONE',  ( 27.87986455999572399, -6.131689368163069531, -3.283357778048667797 ) ) ;
#11894=CARTESIAN_POINT ( 'NONE',  ( 32.97402322492378346, -4.064130265842336165, -3.627061608673664672 ) ) ;
#11899=CARTESIAN_POINT ( 'NONE',  ( 30.61929490284659394, -6.528548903775525325, -4.533357778048668685 ) ) ;
#11905=CARTESIAN_POINT ( 'NONE',  ( 38.64694918415791136, -1.054552983374777098, -1.783357778048662912 ) ) ;
#11910=CARTESIAN_POINT ( 'NONE',  ( 29.77797860222238313, -3.195249460342344250, -3.627061608673662008 ) ) ;
#11911=CARTESIAN_POINT ( 'NONE',  ( 33.60446413004628141, -3.988174587000466342, -3.627061608673664672 ) ) ;
#11917=ORIENTED_EDGE ( 'NONE', *, *, #9974, .F. ) ;
#11924=CARTESIAN_POINT ( 'NONE',  ( 33.01342578063301403, -4.059383036018435753, -8.283357778048662468 ) ) ;
#11925=ORIENTED_EDGE ( 'NONE', *, *, #12421, .F. ) ;
#11930=CARTESIAN_POINT ( 'NONE',  ( 32.12473870642251939, -5.420393343910986594, -7.939653947423664704 ) ) ;
#11934=CARTESIAN_POINT ( 'NONE',  ( 28.56093688906631911, -4.595820017735426255, -3.627061608673664672 ) ) ;
#11937=CARTESIAN_POINT ( 'NONE',  ( 32.92339180097568629, -5.524043937428110063, -3.283357778048667797 ) ) ;
#11953=CARTESIAN_POINT ( 'NONE',  ( 29.77044413525282707, -1.932019286686802895, -6.453230759126468818 ) ) ;
#11954=COLOUR_RGB ( '', 0.31764706, 0.68627451, 0.89019608) ;
#11956=CARTESIAN_POINT ( 'NONE',  ( 30.30787278169304244, -6.266260340387784566, -4.705209693361169343 ) ) ;
#11958=CARTESIAN_POINT ( 'NONE',  ( 32.58190297908952004, -5.565186596593329149, -8.283357778048662468 ) ) ;
#11959=CARTESIAN_POINT ( 'NONE',  ( 26.64639396487419987, -2.308405637095112706, -5.783357778048658027 ) ) ;
#11964=CARTESIAN_POINT ( 'NONE',  ( 31.03886041246737548, -3.043338102658604161, -3.627061608673662008 ) ) ;
#11967=LINE ( 'NONE', #5071, #15972 ) ;
#11977=ADVANCED_FACE ( 'NONE', ( #15796, #10425 ), #4723, .F. ) ;
#11982=CARTESIAN_POINT ( 'NONE',  ( 26.13631296615022137, -5.896629108145342357, -3.732065232213778394 ) ) ;
#11985=CARTESIAN_POINT ( 'NONE',  ( 28.78802868011566929, -7.476087111406434893, -5.783357778048669573 ) ) ;
#11986=CARTESIAN_POINT ( 'NONE',  ( 30.88125018618674034, -3.062327022369072171, -3.627061608673662896 ) ) ;
#11988=( BOUNDED_CURVE ( )  B_SPLINE_CURVE ( 2, ( #12368, #17935, #12288, #2499, #1404, #10985, #2847, #4128, #1501 ),
 .UNSPECIFIED., .F., .T. ) 
 B_SPLINE_CURVE_WITH_KNOTS ( ( 3, 2, 2, 2, 3 ),
 ( 0.7500000000000000000, 0.7564102564102563875, 0.7692307692307692735, 0.7820512820512820484, 0.7884615384615384359 ),
 .UNSPECIFIED. ) 
 CURVE ( )  GEOMETRIC_REPRESENTATION_ITEM ( )  RATIONAL_B_SPLINE_CURVE ( ( 0.9330127018922194093, 0.9330127018922194093, 1.000000000000000000, 0.8660254037844387076, 1.000000000000000000, 0.8660254037844387076, 1.000000000000000000, 0.9330127018922194093, 0.9330127018922194093 ) ) 
 REPRESENTATION_ITEM ( '' )  );
#12004=CARTESIAN_POINT ( 'NONE',  ( 31.69574812466957781, -6.726019302751734763, -5.783357778048669573 ) ) ;
#12005=CARTESIAN_POINT ( 'NONE',  ( 33.17547354829333273, -5.293800545841212291, -3.627061608673667781 ) ) ;
#12013=CARTESIAN_POINT ( 'NONE',  ( 32.84384354600314282, -1.561735352540135180, -6.453230759126467042 ) ) ;
#12018=CARTESIAN_POINT ( 'NONE',  ( 31.38469755857769528, -2.374701023479507178, -4.705209693361161349 ) ) ;
#12020=CARTESIAN_POINT ( 'NONE',  ( 31.67744797322171735, -2.039621600994187656, -7.033357778048658027 ) ) ;
#12024=CARTESIAN_POINT ( 'NONE',  ( 32.24155699611449677, -1.634298987580965923, -5.783357778048664244 ) ) ;
#12032=CARTESIAN_POINT ( 'NONE',  ( 41.90164972253716513, -2.988527579590351646, -5.783357778048662468 ) ) ;
#12035=CARTESIAN_POINT ( 'NONE',  ( 28.26310972651430120, -2.123820177930694442, -5.783357778048658027 ) ) ;
#12045=CARTESIAN_POINT ( 'NONE',  ( 31.02146712245815507, -5.553315781884258229, -7.939653947423662927 ) ) ;
#12046=VERTEX_POINT ( 'NONE', #10157 ) ;
#12049=DIRECTION ( 'NONE',  ( -0.1196152422706584506, 0.9928203230275515212, 0.000000000000000000 ) ) ;
#12057=CARTESIAN_POINT ( 'NONE',  ( 29.70732014299206369, -2.276983097582480742, -7.033357778048658027 ) ) ;
#12062=CARTESIAN_POINT ( 'NONE',  ( 26.19644603989335963, -6.395740563884607432, -4.006386918492157889 ) ) ;
#12066=AXIS2_PLACEMENT_3D ( 'NONE', #4207, #16539, #1310 ) ;
#12067=CARTESIAN_POINT ( 'NONE',  ( 31.91459173804835103, -5.445711903524953712, -3.627061608673667781 ) ) ;
#12079=ORIENTED_EDGE ( 'NONE', *, *, #16115, .F. ) ;
#12084=CARTESIAN_POINT ( 'NONE',  ( 30.43486631442457835, -6.877930660435475296, -5.783357778048669573 ) ) ;
#12085=CARTESIAN_POINT ( 'NONE',  ( 26.14456121274580624, -5.685614013951941992, -8.283357778048664244 ) ) ;
#12093=DIRECTION ( 'NONE',  ( -0.1196152422706598106, 0.9928203230275514102, 0.000000000000000000 ) ) ;
#12099=EDGE_CURVE ( 'NONE', #4757, #10267, #5152, .T. ) ;
#12100=CARTESIAN_POINT ( 'NONE',  ( 27.92859066579839222, -3.218191664895003523, -8.283357778048660691 ) ) ;
#12115=EDGE_CURVE ( 'NONE', #15769, #10379, #2069, .T. ) ;
#12129=CARTESIAN_POINT ( 'NONE',  ( 29.56783163384821833, -3.220568019956291383, -7.939653947423660263 ) ) ;
#12130=( BOUNDED_CURVE ( )  B_SPLINE_CURVE ( 2, ( #15411, #2805, #14051, #16425, #13781, #8330, #13863, #6707, #2997 ),
 .UNSPECIFIED., .F., .T. ) 
 B_SPLINE_CURVE_WITH_KNOTS ( ( 3, 2, 2, 2, 3 ),
 ( 0.1730769230769231004, 0.1794871794871794879, 0.1923076923076923184, 0.2051282051282051211, 0.2115384615384615641 ),
 .UNSPECIFIED. ) 
 CURVE ( )  GEOMETRIC_REPRESENTATION_ITEM ( )  RATIONAL_B_SPLINE_CURVE ( ( 0.9330127018922194093, 0.9330127018922196314, 1.000000000000000000, 0.8660254037844387076, 1.000000000000000000, 0.8660254037844387076, 1.000000000000000000, 0.9330127018922190762, 0.9330127018922194093 ) ) 
 REPRESENTATION_ITEM ( '' )  );
#12139=CARTESIAN_POINT ( 'NONE',  ( 32.70264286945147347, -5.350767304972614546, -3.627061608673668225 ) ) ;
#12151=CARTESIAN_POINT ( 'NONE',  ( 28.19013153391124860, -7.158573733970061248, -5.783357778048657138 ) ) ;
#12157=CARTESIAN_POINT ( 'NONE',  ( 38.70301816123731697, -5.700001250565214228, -1.783357778048662690 ) ) ;
#12158=CONICAL_SURFACE ( 'NONE', #15927, 2.001963570546863025, 0.9599310885968768137 ) ;
#12167=EDGE_CURVE ( 'NONE', #11388, #8115, #10770, .T. ) ;
#12173=( GEOMETRIC_REPRESENTATION_CONTEXT ( 3 ) GLOBAL_UNCERTAINTY_ASSIGNED_CONTEXT ( ( #1733 ) ) GLOBAL_UNIT_ASSIGNED_CONTEXT ( ( #3980, #15128, #8238 ) ) REPRESENTATION_CONTEXT ( 'NONE', 'WORKASPACE' ) );
#12178=FACE_OUTER_BOUND ( 'NONE', #1935, .T. ) ;
#12180=CARTESIAN_POINT ( 'NONE',  ( 27.67650891848073158, -3.448435056481901295, -7.939653947423660263 ) ) ;
#12184=VECTOR ( 'NONE', #6889, 1000.000000000000227 ) ;
#12190=AXIS2_PLACEMENT_3D ( 'NONE', #15804, #4813, #14266 ) ;
#12193=DIRECTION ( 'NONE',  ( -0.1196152422706610735, 0.9928203230275511881, 0.000000000000000000 ) ) ;
#12195=CARTESIAN_POINT ( 'NONE',  ( 33.95908713831676096, -3.945449517755638791, -3.283357778048664688 ) ) ;
#12197=VECTOR ( 'NONE', #9323, 999.9999999999998863 ) ;
#12198=EDGE_CURVE ( 'NONE', #2203, #4586, #5426, .T. ) ;
#12199=DIRECTION ( 'NONE',  ( -0.1196152422706624058, 0.9928203230275510771, 0.000000000000000000 ) ) ;
#12225=CARTESIAN_POINT ( 'NONE',  ( 31.98525019727866692, -6.363978266284800789, -7.033357778048666908 ) ) ;
#12235=CARTESIAN_POINT ( 'NONE',  ( 29.52399153675929355, -1.971908820246954130, -5.783357778048658915 ) ) ;
#12247=CARTESIAN_POINT ( 'NONE',  ( 33.50243880635947846, -1.482387629897225390, -5.783357778048663356 ) ) ;
#12251=LINE ( 'NONE', #11041, #6424 ) ;
#12261=CARTESIAN_POINT ( 'NONE',  ( 29.64681518302145946, -6.972875258987813574, -5.783357778048668685 ) ) ;
#12269=CARTESIAN_POINT ( 'NONE',  ( 33.95908713831674675, -3.945449517755637903, -5.783357778048663356 ) ) ;
#12277=CARTESIAN_POINT ( 'NONE',  ( 33.69269431359690969, -6.158264969628857166, -4.533357778048668685 ) ) ;
#12280=ORIENTED_EDGE ( 'NONE', *, *, #785, .T. ) ;
#12286=LINE ( 'NONE', #13646, #1839 ) ;
#12288=CARTESIAN_POINT ( 'NONE',  ( 28.01872616749444944, -6.841866079205687790, -4.533357778048668685 ) ) ;
#12301=LINE ( 'NONE', #2692, #8933 ) ;
#12302=DIRECTION ( 'NONE',  ( -0.05980762113533058533, 0.4964101615137755386, 0.8660254037844385966 ) ) ;
#12307=CARTESIAN_POINT ( 'NONE',  ( 28.67914455963771303, -4.581578327848842669, -8.283357778048662468 ) ) ;
#12313=( BOUNDED_CURVE ( )  B_SPLINE_CURVE ( 2, ( #2370, #11772, #14516, #3444, #9069, #8974, #4793, #15781, #11959 ),
 .UNSPECIFIED., .F., .T. ) 
 B_SPLINE_CURVE_WITH_KNOTS ( ( 3, 2, 2, 2, 3 ),
 ( 0.7500000000000000000, 0.7564102564102563875, 0.7692307692307692735, 0.7820512820512820484, 0.7884615384615384359 ),
 .UNSPECIFIED. ) 
 CURVE ( )  GEOMETRIC_REPRESENTATION_ITEM ( )  RATIONAL_B_SPLINE_CURVE ( ( 0.9330127018922194093, 0.9330127018922194093, 1.000000000000000000, 0.8660254037844387076, 1.000000000000000000, 0.8660254037844387076, 1.000000000000000000, 0.9330127018922194093, 0.9330127018922194093 ) ) 
 REPRESENTATION_ITEM ( '' )  );
#12314=CARTESIAN_POINT ( 'NONE',  ( 29.78612525785423060, -2.267488637519798012, -7.033357778048658027 ) ) ;
#12316=EDGE_CURVE ( 'NONE', #8115, #17584, #320, .T. ) ;
#12319=FILL_AREA_STYLE ('',( #6963 ) ) ;
#12321=CARTESIAN_POINT ( 'NONE',  ( 28.08810621022444920, -4.652786776866828511, -3.627061608673664672 ) ) ;
#12331=CARTESIAN_POINT ( 'NONE',  ( 28.12741954877813555, -2.767138697495831856, -6.861505862736159145 ) ) ;
#12343=CARTESIAN_POINT ( 'NONE',  ( 28.88938074516742205, -6.437160617781993999, -4.705209693361168455 ) ) ;
#12356=CARTESIAN_POINT ( 'NONE',  ( 28.40332666278570173, -4.614808937445885384, -7.939653947423662039 ) ) ;
#12359=ORIENTED_EDGE ( 'NONE', *, *, #14347, .F. ) ;
#12368=CARTESIAN_POINT ( 'NONE',  ( 28.11132641904908169, -7.168068194032743534, -5.783357778048668685 ) ) ;
#12393=CARTESIAN_POINT ( 'NONE',  ( 26.31128205117621022, -7.047579375861630524, -7.033357778048666908 ) ) ;
#12395=EDGE_CURVE ( 'NONE', #6479, #2500, #9665, .T. ) ;
#12396=CARTESIAN_POINT ( 'NONE',  ( 29.75233713454258933, -1.544652646670201523, -5.783357778048658027 ) ) ;
#12397=DIRECTION ( 'NONE',  ( 0.9928203230275510771, 0.1196152422706609902, 4.006172263299092517E-17 ) ) ;
#12403=CARTESIAN_POINT ( 'NONE',  ( 27.04606801335823718, -3.524390735323771118, -7.939653947423660263 ) ) ;
#12412=CARTESIAN_POINT ( 'NONE',  ( 38.97925773053390941, -7.992821573592766349, -5.783357778048662468 ) ) ;
#12415=CARTESIAN_POINT ( 'NONE',  ( 29.41022140756759029, -3.239556939666760726, -7.939653947423660263 ) ) ;
#12416=CARTESIAN_POINT ( 'NONE',  ( 26.69778786461289855, -6.274106265784127778, -3.283357778048667797 ) ) ;
#12421=EDGE_CURVE ( 'NONE', #16561, #82, #8519, .T. ) ;
#12428=CARTESIAN_POINT ( 'NONE',  ( 28.77978050244509944, -3.315512618508630549, -7.939653947423660263 ) ) ;
#12431=VERTEX_POINT ( 'NONE', #1361 ) ;
#12448=CARTESIAN_POINT ( 'NONE',  ( 26.82722439997946395, -4.804698134550569044, -3.627061608673664672 ) ) ;
#12456=LINE ( 'NONE', #4028, #16209 ) ;
#12464=DIRECTION ( 'NONE',  ( 0.9928203230275512992, 0.1196152422706610319, 9.614813431917826478E-17 ) ) ;
#12477=ORIENTED_EDGE ( 'NONE', *, *, #11072, .T. ) ;
#12483=VECTOR ( 'NONE', #3708, 1000.000000000000114 ) ;
#12486=CARTESIAN_POINT ( 'NONE',  ( 27.14244485254070938, -4.766720295129625029, -7.939653947423662039 ) ) ;
#12489=CARTESIAN_POINT ( 'NONE',  ( 29.26075783691881682, -2.330785036554694489, -4.533357778048659803 ) ) ;
#12493=( NAMED_UNIT ( * ) SI_UNIT ( $, .STERADIAN. ) SOLID_ANGLE_UNIT ( ) );
#12494=CARTESIAN_POINT ( 'NONE',  ( 30.23341599105502908, -5.648260380436597394, -7.939653947423664704 ) ) ;
#12498=CARTESIAN_POINT ( 'NONE',  ( 30.17635249042624679, -2.520282741259753045, -6.861505862736158257 ) ) ;
#12503=ORIENTED_EDGE ( 'NONE', *, *, #8089, .T. ) ;
#12504=ORIENTED_EDGE ( 'NONE', *, *, #12167, .F. ) ;
#12510=CARTESIAN_POINT ( 'NONE',  ( 30.27725608814395031, -6.896919580145944195, -5.783357778048668685 ) ) ;
#12512=FACE_OUTER_BOUND ( 'NONE', #4074, .T. ) ;
#12523=CARTESIAN_POINT ( 'NONE',  ( 26.97161122272022382, -2.906390775372597712, -4.705209693361161349 ) ) ;
#12525=DIRECTION ( 'NONE',  ( 0.9928203230275512992, 0.1196152422706610180, 4.006172263299093133E-17 ) ) ;
#12530=AXIS2_PLACEMENT_3D ( 'NONE', #3329, #16847, #14113 ) ;
#12534=VERTEX_POINT ( 'NONE', #6432 ) ;
#12540=CARTESIAN_POINT ( 'NONE',  ( 31.80137159822941939, -6.386132006154467078, -4.533357778048668685 ) ) ;
#12550=( LENGTH_UNIT ( ) NAMED_UNIT ( * ) SI_UNIT ( .MILLI., .METRE. ) );
#12559=PRODUCT_CONTEXT ( 'NONE', #10804, 'mechanical' ) ;
#12574=ORIENTED_EDGE ( 'NONE', *, *, #14226, .T. ) ;
#12579=CARTESIAN_POINT ( 'NONE',  ( 25.93489015466116854, -5.606035894254070229, -7.939653947423662927 ) ) ;
#12581=CARTESIAN_POINT ( 'NONE',  ( 33.53059316159333036, -1.478995586096186532, -5.113484796970854340 ) ) ;
#12582=ORIENTED_EDGE ( 'NONE', *, *, #5265, .T. ) ;
#12583=CARTESIAN_POINT ( 'NONE',  ( 27.86101441917510257, -1.772519683195811657, -5.783357778048658027 ) ) ;
#12587=CARTESIAN_POINT ( 'NONE',  ( 31.38469755857769528, -2.374701023479507178, -4.705209693361161349 ) ) ;
#12589=CARTESIAN_POINT ( 'NONE',  ( 30.43486631442457835, -6.877930660435475296, -5.783357778048669573 ) ) ;
#12601=CARTESIAN_POINT ( 'NONE',  ( 30.86385689617752348, -5.572304701594726239, -7.939653947423664704 ) ) ;
#12603=CARTESIAN_POINT ( 'NONE',  ( 39.40660799972354056, -7.359808871700536770, -5.783357778048663356 ) ) ;
#12614=CARTESIAN_POINT ( 'NONE',  ( 30.04066231269008469, -3.163601260824890904, -7.939653947423660263 ) ) ;
#12628=CARTESIAN_POINT ( 'NONE',  ( 31.00199007654869732, -2.847907730748336252, -8.283357778048658915 ) ) ;
#12632=CARTESIAN_POINT ( 'NONE',  ( 46.86575133767495061, -2.390451368237048069, -5.783357778048661579 ) ) ;
#12635=EDGE_LOOP ( 'NONE', ( #7708, #15339, #16767, #5378 ) ) ;
#12654=CARTESIAN_POINT ( 'NONE',  ( 31.68992120585416217, -1.700760206360153015, -5.783357778048664244 ) ) ;
#12663=CARTESIAN_POINT ( 'NONE',  ( 28.36392410707646761, -4.619556167269785796, -3.283357778048664688 ) ) ;
#12664=VECTOR ( 'NONE', #14327, 1000.000000000000227 ) ;
#12667=CARTESIAN_POINT ( 'NONE',  ( 31.27962407439061110, -2.387360303286481855, -6.861505862736159145 ) ) ;
#12670=CARTESIAN_POINT ( 'NONE',  ( 27.28266178881210280, -7.257709054644825741, -5.783357778048669573 ) ) ;
#12681=CARTESIAN_POINT ( 'NONE',  ( 28.53771668024168662, -2.080538600569502794, -5.783357778048658027 ) ) ;
#12682=CARTESIAN_POINT ( 'NONE',  ( 28.88938074516742205, -6.437160617781993999, -4.705209693361168455 ) ) ;
#12690=AXIS2_PLACEMENT_3D ( 'NONE', #9473, #17783, #2599 ) ;
#12700=EDGE_CURVE ( 'NONE', #17201, #13578, #1529, .T. ) ;
#12701=DIRECTION ( 'NONE',  ( 0.000000000000000000, -0.5027044994213120122, -0.8644583195629319539 ) ) ;
#12712=CARTESIAN_POINT ( 'NONE',  ( 31.30979230060565044, -7.172264396038955603, -5.783357778048669573 ) ) ;
#12726=CARTESIAN_POINT ( 'NONE',  ( 38.15053902264412500, -1.114360604510109765, -9.783357778048662468 ) ) ;
#12735=CARTESIAN_POINT ( 'NONE',  ( 32.29974222271236073, -2.891426744974864071, -3.627061608673662008 ) ) ;
#12737=DIRECTION ( 'NONE',  ( -0.9928203230275512992, -0.1196152422706610319, -9.614813431917826478E-17 ) ) ;
#12740=CLOSED_SHELL ( 'NONE', ( #17156, #8212, #7574, #15108, #5369, #2417, #3945, #16991, #4766, #17044, #1905, #8185, #2697, #3744, #465, #15842, #7735, #3209, #13358, #3027, #389, #9794, #8013, #5549, #2401, #5911, #13949, #7374, #16082, #14983, #3844, #9371, #13133, #17062, #7320, #16317, #7535, #17168, #11977, #444, #10694, #14013, #365, #7373, #1969, #14431, #12797, #13182, #8005, #5090, #8278, #10760, #15653, #17796, #13034, #15466, #16704 ) ) ;
#12741=ORIENTED_EDGE ( 'NONE', *, *, #17889, .F. ) ;
#12751=FACE_OUTER_BOUND ( 'NONE', #12635, .T. ) ;
#12754=CARTESIAN_POINT ( 'NONE',  ( 26.32044349065828115, -7.243571858916999950, -6.694428052743685242 ) ) ;
#12757=CARTESIAN_POINT ( 'NONE',  ( 26.94172295629870462, -6.971623697019761146, -7.033357778048666908 ) ) ;
#12761=CARTESIAN_POINT ( 'NONE',  ( 30.27725608814395031, -6.896919580145944195, -5.783357778048668685 ) ) ;
#12763=CARTESIAN_POINT ( 'NONE',  ( 25.88432464927661769, -3.805096980563277498, -7.814840548041910750 ) ) ;
#12771=PLANE ( 'NONE',  #14297 ) ;
#12772=CARTESIAN_POINT ( 'NONE',  ( 46.86575133767495061, -2.390451368237048069, -5.783357778048661579 ) ) ;
#12776=CARTESIAN_POINT ( 'NONE',  ( 32.80318959510331212, -2.203800746085299522, -4.705209693361160461 ) ) ;
#12783=ORIENTED_EDGE ( 'NONE', *, *, #4556, .F. ) ;
#12790=CARTESIAN_POINT ( 'NONE',  ( 26.34117031759772942, -2.982346454214467535, -4.705209693361161349 ) ) ;
#12797=ADVANCED_FACE ( 'NONE', ( #11100 ), #16668, .T. ) ;
#12804=FACE_OUTER_BOUND ( 'NONE', #11370, .T. ) ;
#12809=CARTESIAN_POINT ( 'NONE',  ( 30.44283453230164227, -2.188368138933637574, -4.533357778048659803 ) ) ;
#12810=VECTOR ( 'NONE', #12397, 1000.000000000000227 ) ;
#12845=CARTESIAN_POINT ( 'NONE',  ( 32.37175601071535169, -5.590505156207296267, -3.283357778048667797 ) ) ;
#12850=PLANE ( 'NONE',  #11263 ) ;
#12856=CARTESIAN_POINT ( 'NONE',  ( 33.19286683830256379, -2.783822866615540903, -7.939653947423660263 ) ) ;
#12857=LINE ( 'NONE', #7339, #8957 ) ;
#12861=CARTESIAN_POINT ( 'NONE',  ( 31.93198502805756789, -2.935734224299280548, -7.939653947423660263 ) ) ;
#12875=CARTESIAN_POINT ( 'NONE',  ( 32.08959525433819238, -2.916745304588811649, -7.939653947423660263 ) ) ;
#12878=CARTESIAN_POINT ( 'NONE',  ( 27.81599742762458050, -2.504850134108091098, -7.033357778048658027 ) ) ;
#12884=PLANE ( 'NONE',  #823 ) ;
#12887=DIRECTION ( 'NONE',  ( -0.1196152422706610735, 0.9928203230275511881, 0.000000000000000000 ) ) ;
#12888=ORIENTED_EDGE ( 'NONE', *, *, #12316, .F. ) ;
#12892=CARTESIAN_POINT ( 'NONE',  ( 29.32081432955537537, -3.050456207659999475, -3.283357778048662023 ) ) ;
#12894=EDGE_LOOP ( 'NONE', ( #1720, #16824, #14667, #4291, #10794, #6781, #11113, #6219, #5244, #16699, #17328, #12888, #2871, #13136, #5091, #9393, #10104, #3284, #890, #7827, #5447, #6124, #641, #7760, #609, #16545, #414, #38 ) ) ;
#12896=CARTESIAN_POINT ( 'NONE',  ( 26.70901672940806648, -4.818939824437135755, -8.283357778048662468 ) ) ;
#12897=( BOUNDED_CURVE ( )  B_SPLINE_CURVE ( 2, ( #11435, #8829, #3200, #8642, #15725, #1762, #14452, #8742, #1860 ),
 .UNSPECIFIED., .F., .T. ) 
 B_SPLINE_CURVE_WITH_KNOTS ( ( 3, 2, 2, 2, 3 ),
 ( 0.5576923076923077094, 0.5641025641025640969, 0.5769230769230768718, 0.5897435897435897578, 0.5961538461538461453 ),
 .UNSPECIFIED. ) 
 CURVE ( )  GEOMETRIC_REPRESENTATION_ITEM ( )  RATIONAL_B_SPLINE_CURVE ( ( 0.9330127018922194093, 0.9330127018922194093, 1.000000000000000000, 0.8660254037844387076, 1.000000000000000000, 0.8660254037844387076, 1.000000000000000000, 0.9330127018922194093, 0.9330127018922194093 ) ) 
 REPRESENTATION_ITEM ( '' )  );
#12902=CARTESIAN_POINT ( 'NONE',  ( 30.61177514885987350, -5.802548093181622235, -8.283357778048662468 ) ) ;
#12904=EDGE_CURVE ( 'NONE', #397, #2657, #1110, .T. ) ;
#12918=CARTESIAN_POINT ( 'NONE',  ( 33.46007730730551799, -5.886481946178435010, -4.705209693361169343 ) ) ;
#12919=DIRECTION ( 'NONE',  ( 0.05980762113533198004, -0.4964101615137755941, 0.8660254037844384856 ) ) ;
#12928=CARTESIAN_POINT ( 'NONE',  ( 31.78252145740879797, -2.026962321187214311, -4.533357778048659803 ) ) ;
#12933=DIRECTION ( 'NONE',  ( 0.1035898384862230237, -0.8598076211353317122, -0.5000000000000002220 ) ) ;
#12938=CARTESIAN_POINT ( 'NONE',  ( 26.24741491880507027, -3.420740141806666745, -3.283357778048662023 ) ) ;
#12941=CARTESIAN_POINT ( 'NONE',  ( 27.08121146544255353, -6.028038774645947839, -7.939653947423664704 ) ) ;
#12943=CARTESIAN_POINT ( 'NONE',  ( 26.18940075748478691, -6.337263906362392341, -7.823530922983556124 ) ) ;
#12950=CARTESIAN_POINT ( 'NONE',  ( 26.92924972366625980, -7.310485091653801781, -5.783357778048657138 ) ) ;
#12957=CARTESIAN_POINT ( 'NONE',  ( 31.87075164095941915, -4.197052703815608687, -3.627061608673664672 ) ) ;
#12959=DIRECTION ( 'NONE',  ( 0.9928203230275512992, 0.1196152422706610180, 4.006172263299093133E-17 ) ) ;
#12966=CARTESIAN_POINT ( 'NONE',  ( 30.52163964716380917, -2.178873678870954400, -4.533357778048659803 ) ) ;
#12989=CARTESIAN_POINT ( 'NONE',  ( 30.04891049036066164, -7.324175753722694360, -5.783357778048669573 ) ) ;
#12993=ORIENTED_EDGE ( 'NONE', *, *, #10180, .T. ) ;
#12998=DIRECTION ( 'NONE',  ( 0.9928203230275510771, 0.1196152422706609902, 4.006172263299092517E-17 ) ) ;
#13007=DIRECTION ( 'NONE',  ( -0.1196152422706610735, 0.9928203230275511881, 0.000000000000000000 ) ) ;
#13016=CARTESIAN_POINT ( 'NONE',  ( 39.22222685913116180, -5.829424113971213295, -5.783357778048662468 ) ) ;
#13017=ORIENTED_EDGE ( 'NONE', *, *, #1913, .T. ) ;
#13020=CARTESIAN_POINT ( 'NONE',  ( 27.18555652250208610, -2.580805812949960920, -7.033357778048658027 ) ) ;
#13025=CARTESIAN_POINT ( 'NONE',  ( 25.29083129957448151, -4.989803161779970964, -5.783357778048664244 ) ) ;
#13027=CARTESIAN_POINT ( 'NONE',  ( 26.00347982711925710, -2.723222710571018279, -7.033357778048658027 ) ) ;
#13028=EDGE_CURVE ( 'NONE', #6811, #3520, #9110, .T. ) ;
#13031=CARTESIAN_POINT ( 'NONE',  ( 26.34117031759772942, -2.982346454214467535, -4.705209693361161349 ) ) ;
#13034=ADVANCED_FACE ( 'NONE', ( #4575 ), #5278, .T. ) ;
#13035=CARTESIAN_POINT ( 'NONE',  ( 26.08205926866327218, -5.446317154234562530, -8.158109112226842541 ) ) ;
#13037=ORIENTED_EDGE ( 'NONE', *, *, #1345, .T. ) ;
#13047=CARTESIAN_POINT ( 'NONE',  ( 32.81641299864316608, -4.083119185552795294, -7.939653947423662039 ) ) ;
#13050=ORIENTED_EDGE ( 'NONE', *, *, #10386, .F. ) ;
#13070=CARTESIAN_POINT ( 'NONE',  ( 30.00264913441657555, -6.940201157507134511, -5.783357778048657138 ) ) ;
#13083=CARTESIAN_POINT ( 'NONE',  ( 27.81599742762458050, -2.504850134108091098, -7.033357778048658027 ) ) ;
#13089=EDGE_CURVE ( 'NONE', #7189, #13433, #2650, .T. ) ;
#13091=CARTESIAN_POINT ( 'NONE',  ( 30.72436838703367812, -6.515889623968540434, -7.033357778048666908 ) ) ;
#13097=CARTESIAN_POINT ( 'NONE',  ( 25.92409770820621162, -4.135217962343409326, -3.765474553462066165 ) ) ;
#13107=CARTESIAN_POINT ( 'NONE',  ( 31.56875459193803124, -6.114348982704044921, -4.705209693361169343 ) ) ;
#13113=CARTESIAN_POINT ( 'NONE',  ( 26.45077056032005913, -6.103994453487816330, -7.939653947423664704 ) ) ;
#13114=ORIENTED_EDGE ( 'NONE', *, *, #3823, .F. ) ;
#13122=CARTESIAN_POINT ( 'NONE',  ( 27.87912141988533676, -2.159886323212414361, -6.453230759126469707 ) ) ;
#13125=CARTESIAN_POINT ( 'NONE',  ( 26.47260139170898441, -4.847423203795396596, -3.283357778048664688 ) ) ;
#13127=DIRECTION ( 'NONE',  ( 0.000000000000000000, -0.5027044994213123452, 0.8644583195629317318 ) ) ;
#13129=CARTESIAN_POINT ( 'NONE',  ( 29.50659824675005893, -4.481886499472614638, -7.939653947423662039 ) ) ;
#13133=ADVANCED_FACE ( 'NONE', ( #6899 ), #2397, .F. ) ;
#13136=ORIENTED_EDGE ( 'NONE', *, *, #1038, .F. ) ;
#13140=CARTESIAN_POINT ( 'NONE',  ( 29.16815758536418102, -2.004582921727632971, -5.783357778048664244 ) ) ;
#13142=CARTESIAN_POINT ( 'NONE',  ( 32.69811611091622439, -2.216460025892273311, -6.861505862736158257 ) ) ;
#13152=CARTESIAN_POINT ( 'NONE',  ( 32.30426898124760982, -6.025734024055190652, -6.861505862736167138 ) ) ;
#13160=ORIENTED_EDGE ( 'NONE', *, *, #15391, .T. ) ;
#13163=CARTESIAN_POINT ( 'NONE',  ( 33.00465954875439678, 3.976409685033599484, 3.995355914169179040E-15 ) ) ;
#13164=CARTESIAN_POINT ( 'NONE',  ( 33.50243880635947846, -1.482387629897225390, -5.783357778048663356 ) ) ;
#13165=EDGE_CURVE ( 'NONE', #8339, #17201, #17728, .T. ) ;
#13166=CARTESIAN_POINT ( 'NONE',  ( 27.27683486999669427, -2.232449958253242883, -5.783357778048658027 ) ) ;
#13167=( BOUNDED_CURVE ( )  B_SPLINE_CURVE ( 2, ( #17542, #17083, #15801, #3194, #12896, #4638, #8822, #14784, #3810 ),
 .UNSPECIFIED., .F., .T. ) 
 B_SPLINE_CURVE_WITH_KNOTS ( ( 3, 2, 2, 2, 3 ),
 ( 0.8653846153846154188, 0.8717948717948718063, 0.8846153846153845812, 0.8974358974358974672, 0.9038461538461538547 ),
 .UNSPECIFIED. ) 
 CURVE ( )  GEOMETRIC_REPRESENTATION_ITEM ( )  RATIONAL_B_SPLINE_CURVE ( ( 0.9330127018922192983, 0.9330127018922198534, 1.000000000000000000, 0.8660254037844387076, 1.000000000000000000, 0.8660254037844387076, 1.000000000000000000, 0.9330127018922194093, 0.9330127018922194093 ) ) 
 REPRESENTATION_ITEM ( '' )  );
#13175=CARTESIAN_POINT ( 'NONE',  ( 27.96989853965305528, -4.667028466753395222, -8.283357778048662468 ) ) ;
#13177=EDGE_CURVE ( 'NONE', #14372, #15406, #13272, .T. ) ;
#13182=ADVANCED_FACE ( 'NONE', ( #11218 ), #12884, .T. ) ;
#13191=FACE_OUTER_BOUND ( 'NONE', #1902, .T. ) ;
#13194=CARTESIAN_POINT ( 'NONE',  ( 29.66420847303068697, -4.462897579762144851, -7.939653947423662039 ) ) ;
#13195=LINE ( 'NONE', #10279, #13980 ) ;
#13212=CARTESIAN_POINT ( 'NONE',  ( 32.34358231980129261, -4.140085944684206432, -3.627061608673664672 ) ) ;
#13217=CARTESIAN_POINT ( 'NONE',  ( 28.87615734162756453, -4.557842178314484016, -7.939653947423662039 ) ) ;
#13220=VERTEX_POINT ( 'NONE', #5701 ) ;
#13226=CARTESIAN_POINT ( 'NONE',  ( 29.46348657678868577, -6.667800981652280967, -7.033357778048666908 ) ) ;
#13228=CARTESIAN_POINT ( 'NONE',  ( 30.93831368681553684, -6.190304661545915188, -4.705209693361169343 ) ) ;
#13231=CARTESIAN_POINT ( 'NONE',  ( 32.30788887834420819, -1.963665922152317833, -7.033357778048658027 ) ) ;
#13232=CARTESIAN_POINT ( 'NONE',  ( 31.37049041475757605, -6.775403295959669947, -6.453230759126470595 ) ) ;
#13237=CARTESIAN_POINT ( 'NONE',  ( 30.80679339554874119, -2.444327062417882779, -6.861505862736158257 ) ) ;
#13241=VECTOR ( 'NONE', #11146, 1000.000000000000114 ) ;
#13252=VECTOR ( 'NONE', #2031, 1000.000000000000227 ) ;
#13255=CARTESIAN_POINT ( 'NONE',  ( 26.28374211850152875, -7.120308096563231715, -4.880631602441031447 ) ) ;
#13257=DIRECTION ( 'NONE',  ( 0.9928203230275512992, 0.1196152422706610735, 9.614813431917828943E-17 ) ) ;
#13258=CARTESIAN_POINT ( 'NONE',  ( 28.91555989733679866, -4.553094948490599592, -3.283357778048664688 ) ) ;
#13259=CARTESIAN_POINT ( 'NONE',  ( 32.14213199643173624, -2.910415664685331638, -3.627061608673662896 ) ) ;
#13269=CARTESIAN_POINT ( 'NONE',  ( 30.98067518586950442, -1.786210345264705790, -5.783357778048658027 ) ) ;
#13271=FACE_OUTER_BOUND ( 'NONE', #10181, .T. ) ;
#13272=CIRCLE ( 'NONE', #2834, 3.425051884552432035 ) ;
#13273=EDGE_CURVE ( 'NONE', #12431, #15406, #17072, .T. ) ;
#13280=CARTESIAN_POINT ( 'NONE',  ( 30.15443244188179150, -1.895953141405084086, -5.783357778048658027 ) ) ;
#13281=FACE_OUTER_BOUND ( 'NONE', #11789, .T. ) ;
#13293=CARTESIAN_POINT ( 'NONE',  ( 32.85952466860454280, -1.897204703373130741, -7.033357778048658027 ) ) ;
#13296=CYLINDRICAL_SURFACE ( 'NONE', #4125, 2.500000000000001776 ) ;
#13299=CARTESIAN_POINT ( 'NONE',  ( 31.28415083292585663, -5.521667582366822202, -3.627061608673667781 ) ) ;
#13302=CARTESIAN_POINT ( 'NONE',  ( 27.09860475545177039, -3.518061095420291995, -3.627061608673662896 ) ) ;
#13306=DIRECTION ( 'NONE',  ( 0.9928203230275510771, 0.1196152422706609902, 4.006172263299092517E-17 ) ) ;
#13319=CARTESIAN_POINT ( 'NONE',  ( 29.42969845347704450, -5.944964990802679594, -8.283357778048664244 ) ) ;
#13321=CARTESIAN_POINT ( 'NONE',  ( 27.75966235412334981, -2.811446176820259879, -4.705209693361160461 ) ) ;
#13326=CARTESIAN_POINT ( 'NONE',  ( 31.03132594549780876, -1.780107929003061473, -6.453230759126465266 ) ) ;
#13327=EDGE_CURVE ( 'NONE', #4586, #2990, #4799, .T. ) ;
#13331=CARTESIAN_POINT ( 'NONE',  ( 31.04338717100262102, -6.177645381738930297, -6.861505862736167138 ) ) ;
#13354=CARTESIAN_POINT ( 'NONE',  ( 33.81344892038539740, -6.481075040654872943, -6.453230759126470595 ) ) ;
#13355=CARTESIAN_POINT ( 'NONE',  ( 27.24942365487322959, -6.207645047004941574, -3.283357778048667797 ) ) ;
#13356=CARTESIAN_POINT ( 'NONE',  ( 31.27962407439061110, -2.387360303286481855, -6.861505862736159145 ) ) ;
#13358=ADVANCED_FACE ( 'NONE', ( #17549 ), #555, .T. ) ;
#13373=CARTESIAN_POINT ( 'NONE',  ( 29.03376756790819613, -4.538853258604016006, -7.939653947423662039 ) ) ;
#13374=VECTOR ( 'NONE', #4882, 1000.000000000000000 ) ;
#13375=CARTESIAN_POINT ( 'NONE',  ( 33.17094678975809074, -2.159493266760871499, -6.861505862736159145 ) ) ;
#13387=DIRECTION ( 'NONE',  ( 0.05980762113533047430, -0.4964101615137755941, -0.8660254037844387076 ) ) ;
#13395=CARTESIAN_POINT ( 'NONE',  ( 31.93198502805756789, -2.935734224299280548, -7.939653947423660263 ) ) ;
#13396=CARTESIAN_POINT ( 'NONE',  ( 38.64694918415791136, -1.054552983374777986, -9.783357778048662468 ) ) ;
#13397=CARTESIAN_POINT ( 'NONE',  ( 31.97277696464621854, -6.702839660918840536, -5.783357778048663356 ) ) ;
#13415=( GEOMETRIC_REPRESENTATION_CONTEXT ( 3 ) GLOBAL_UNCERTAINTY_ASSIGNED_CONTEXT ( ( #5338 ) ) GLOBAL_UNIT_ASSIGNED_CONTEXT ( ( #12550, #2942, #15265 ) ) REPRESENTATION_CONTEXT ( 'NONE', 'WORKASPACE' ) );
#13417=CARTESIAN_POINT ( 'NONE',  ( 28.91999743871649997, -5.806501378023834370, -3.627061608673668225 ) ) ;
#13421=CARTESIAN_POINT ( 'NONE',  ( 31.71123609653335507, -2.762457591843783256, -8.283357778048658915 ) ) ;
#13429=CARTESIAN_POINT ( 'NONE',  ( 33.43363050022580296, -2.127845067243429256, -4.705209693361160461 ) ) ;
#13433=VERTEX_POINT ( 'NONE', #10511 ) ;
#13437=CARTESIAN_POINT ( 'NONE',  ( 28.64916707261694384, -6.765910400363817523, -4.533357778048668685 ) ) ;
#13439=CARTESIAN_POINT ( 'NONE',  ( 33.68284756902015431, -1.652629194728085338, -9.783357778048662468 ) ) ;
#13446=CARTESIAN_POINT ( 'NONE',  ( 33.79776779778399032, -6.145605689821873163, -7.033357778048666908 ) ) ;
#13447=DIRECTION ( 'NONE',  ( 0.000000000000000000, -0.000000000000000000, 1.000000000000000000 ) ) ;
#13448=CARTESIAN_POINT ( 'NONE',  ( 30.65370992780335868, -5.597623261208692469, -3.627061608673667781 ) ) ;
#13471=CARTESIAN_POINT ( 'NONE',  ( 30.93831368681553684, -6.190304661545915188, -4.705209693361169343 ) ) ;
#13481=CARTESIAN_POINT ( 'NONE',  ( 26.31065902414478330, -7.328232685206446106, -6.312034385895062272 ) ) ;
#13487=( BOUNDED_CURVE ( )  B_SPLINE_CURVE ( 2, ( #12151, #6985, #15689, #3089, #7441, #4616, #2899, #5694, #8429 ),
 .UNSPECIFIED., .F., .T. ) 
 B_SPLINE_CURVE_WITH_KNOTS ( ( 3, 2, 2, 2, 3 ),
 ( 0.6730769230769231282, 0.6794871794871795156, 0.6923076923076922906, 0.7051282051282051766, 0.7115384615384615641 ),
 .UNSPECIFIED. ) 
 CURVE ( )  GEOMETRIC_REPRESENTATION_ITEM ( )  RATIONAL_B_SPLINE_CURVE ( ( 0.9330127018922192983, 0.9330127018922198534, 1.000000000000000000, 0.8660254037844387076, 1.000000000000000000, 0.8660254037844387076, 1.000000000000000000, 0.9330127018922194093, 0.9330127018922194093 ) ) 
 REPRESENTATION_ITEM ( '' )  );
#13500=CYLINDRICAL_SURFACE ( 'NONE', #16198, 2.500000000000000000 ) ;
#13501=CARTESIAN_POINT ( 'NONE',  ( 30.10960860451258370, -6.927314653643411368, -6.453230759126470595 ) ) ;
#13503=CARTESIAN_POINT ( 'NONE',  ( 30.41294626588012306, -6.253601060580800564, -6.861505862736167138 ) ) ;
#13514=CARTESIAN_POINT ( 'NONE',  ( 33.46007730730551799, -5.886481946178435010, -4.705209693361169343 ) ) ;
#13530=LINE ( 'NONE', #2303, #9309 ) ;
#13535=CARTESIAN_POINT ( 'NONE',  ( 31.30154412293507349, -3.011689903141150815, -7.939653947423660263 ) ) ;
#13536=ORIENTED_EDGE ( 'NONE', *, *, #7038, .T. ) ;
#13550=CARTESIAN_POINT ( 'NONE',  ( 33.52375369703867847, -2.544085015380856518, -8.283357778048658915 ) ) ;
#13564=CIRCLE ( 'NONE', #6906, 2.705189185291143605 ) ;
#13572=CYLINDRICAL_SURFACE ( 'NONE', #12690, 2.500000000000001776 ) ;
#13578=VERTEX_POINT ( 'NONE', #1088 ) ;
#13581=CARTESIAN_POINT ( 'NONE',  ( 28.50956232500783472, -2.083930644370540985, -6.453230759126464378 ) ) ;
#13586=CARTESIAN_POINT ( 'NONE',  ( 26.31556265977298992, -7.384422263489805793, -5.783357778048663356 ) ) ;
#13588=CARTESIAN_POINT ( 'NONE',  ( 31.02146712245815507, -5.553315781884258229, -7.939653947423664704 ) ) ;
#13591=CARTESIAN_POINT ( 'NONE',  ( 31.92138306490751987, -2.737139032229836122, -3.283357778048662023 ) ) ;
#13597=CARTESIAN_POINT ( 'NONE',  ( 30.39102621733566423, -5.629271460726127607, -7.939653947423662927 ) ) ;
#13615=VERTEX_POINT ( 'NONE', #4431 ) ;
#13622=AXIS2_PLACEMENT_3D ( 'NONE', #17683, #3865, #12193 ) ;
#13623=CARTESIAN_POINT ( 'NONE',  ( 28.99445422935450267, -6.424501337975009996, -6.861505862736166250 ) ) ;
#13636=CARTESIAN_POINT ( 'NONE',  ( 27.89118264539014547, -6.557423775948280742, -6.861505862736167138 ) ) ;
#13639=VECTOR ( 'NONE', #16781, 1000.000000000000227 ) ;
#13646=CARTESIAN_POINT ( 'NONE',  ( 34.23532670761333918, -6.238269840783189579, -1.783357778048662690 ) ) ;
#13668=DIRECTION ( 'NONE',  ( 0.7752790601682274518, -0.5233950504778107637, 0.3535533905932737864 ) ) ;
#13675=CARTESIAN_POINT ( 'NONE',  ( 26.39823381822651882, -6.110324093391315436, -3.627061608673668225 ) ) ;
#13678=CARTESIAN_POINT ( 'NONE',  ( 27.89480254248674740, -2.495355674045408367, -7.033357778048658027 ) ) ;
#13687=CARTESIAN_POINT ( 'NONE',  ( 28.28955653359400557, -5.882457056865704637, -3.627061608673668225 ) ) ;
#13699=CARTESIAN_POINT ( 'NONE',  ( 28.38593337277646711, -7.124786616671554107, -5.783357778048668685 ) ) ;
#13714=CARTESIAN_POINT ( 'NONE',  ( 29.01637427789896151, -7.048830937829682064, -5.783357778048668685 ) ) ;
#13724=CARTESIAN_POINT ( 'NONE',  ( 33.73390066541284682, -2.518766455766909385, -3.283357778048662023 ) ) ;
#13725=EDGE_CURVE ( 'NONE', #12534, #3987, #15143, .T. ) ;
#13726=VERTEX_POINT ( 'NONE', #9456 ) ;
#13755=CARTESIAN_POINT ( 'NONE',  ( 28.52524344760924180, -2.419399995203538101, -7.033357778048658027 ) ) ;
#13762=CARTESIAN_POINT ( 'NONE',  ( 26.15738093914773543, -4.885401043216321959, -8.283357778048662468 ) ) ;
#13764=ORIENTED_EDGE ( 'NONE', *, *, #3519, .T. ) ;
#13765=CARTESIAN_POINT ( 'NONE',  ( 31.35480929215617252, -6.439933945126671055, -7.033357778048666908 ) ) ;
#13769=EDGE_LOOP ( 'NONE', ( #2055, #1924, #3255, #1458 ) ) ;
#13773=CARTESIAN_POINT ( 'NONE',  ( 29.76058531221316272, -5.705227139567997874, -7.939653947423662927 ) ) ;
#13777=ORIENTED_EDGE ( 'NONE', *, *, #5069, .T. ) ;
#13781=CARTESIAN_POINT ( 'NONE',  ( 32.38298487551052318, -4.135338714860305132, -8.283357778048662468 ) ) ;
#13783=CARTESIAN_POINT ( 'NONE',  ( 33.55383270609817714, -5.448088258586239796, -3.283357778048667797 ) ) ;
#13784=CARTESIAN_POINT ( 'NONE',  ( 27.47505859511117521, -2.218764776483033163, -5.783357778048658027 ) ) ;
#13795=CARTESIAN_POINT ( 'NONE',  ( 27.49697864365563760, -2.843094376337701679, -6.861505862736159145 ) ) ;
#13806=DIRECTION ( 'NONE',  ( 0.9928203230275510771, 0.1196152422706609902, 4.006172263299092517E-17 ) ) ;
#13807=CARTESIAN_POINT ( 'NONE',  ( 27.91310269393460430, -7.181753375802955475, -5.783357778048669573 ) ) ;
#13816=EDGE_LOOP ( 'NONE', ( #2964, #12574, #5775, #3286 ) ) ;
#13835=VERTEX_POINT ( 'NONE', #8383 ) ;
#13842=CARTESIAN_POINT ( 'NONE',  ( 25.71748644841968456, -2.420320648352046078, -5.783357778048663356 ) ) ;
#13844=CARTESIAN_POINT ( 'NONE',  ( 25.78518620311324838, -3.676302093007511651, -7.939653947423660263 ) ) ;
#13846=CARTESIAN_POINT ( 'NONE',  ( 30.06013935859953534, -5.869009311960810216, -8.283357778048662468 ) ) ;
#13851=CARTESIAN_POINT ( 'NONE',  ( 29.04699097144805364, -6.418171698071525100, -4.705209693361169343 ) ) ;
#13863=CARTESIAN_POINT ( 'NONE',  ( 32.53688598753899441, -6.297517047505613697, -7.033357778048666908 ) ) ;
#13866=CARTESIAN_POINT ( 'NONE',  ( 29.62036837594175154, -3.214238380052812261, -3.627061608673662896 ) ) ;
#13869=FACE_BOUND ( 'NONE', #1933, .T. ) ;
#13877=CARTESIAN_POINT ( 'NONE',  ( 42.73333828282231650, -6.338146013849483396, -5.783357778048662468 ) ) ;
#13880=CARTESIAN_POINT ( 'NONE',  ( 28.25893984004492765, -6.513116296623863377, -4.705209693361168455 ) ) ;
#13894=CARTESIAN_POINT ( 'NONE',  ( 26.52522735095806894, -6.721994413439005278, -4.705209693361169343 ) ) ;
#13906=EDGE_LOOP ( 'NONE', ( #17767, #16790, #2433, #12079, #8792, #2243 ) ) ;
#13923=VERTEX_POINT ( 'NONE', #11543 ) ;
#13934=CARTESIAN_POINT ( 'NONE',  ( 37.96876116389215383, 4.574485896386907058, -2.283357778048670461 ) ) ;
#13935=CARTESIAN_POINT ( 'NONE',  ( 26.51200394741821498, -4.842675973971495296, -7.939653947423662039 ) ) ;
#13938=CARTESIAN_POINT ( 'NONE',  ( 28.86683379497783264, -7.466592651343750831, -5.783357778048669573 ) ) ;
#13942=CARTESIAN_POINT ( 'NONE',  ( 32.67202617590239555, -5.981426544730773287, -4.705209693361168455 ) ) ;
#13945=CARTESIAN_POINT ( 'NONE',  ( 29.14753769709988518, -3.271205139184214072, -3.627061608673662008 ) ) ;
#13946=EDGE_LOOP ( 'NONE', ( #9331, #8950, #2918, #1067 ) ) ;
#13949=ADVANCED_FACE ( 'NONE', ( #2150 ), #14652, .T. ) ;
#13951=( BOUNDED_CURVE ( )  B_SPLINE_CURVE ( 2, ( #10205, #16940, #1974, #5663, #15381, #1613, #1797, #10013, #15474 ),
 .UNSPECIFIED., .F., .T. ) 
 B_SPLINE_CURVE_WITH_KNOTS ( ( 3, 2, 2, 2, 3 ),
 ( 0.2115384615384615641, 0.2179487179487179516, 0.2307692307692307820, 0.2435897435897435848, 0.2500000000000000000 ),
 .UNSPECIFIED. ) 
 CURVE ( )  GEOMETRIC_REPRESENTATION_ITEM ( )  RATIONAL_B_SPLINE_CURVE ( ( 0.9330127018922194093, 0.9330127018922196314, 1.000000000000000000, 0.8660254037844387076, 1.000000000000000000, 0.8660254037844387076, 1.000000000000000000, 0.9330127018922191873, 0.9330127018922194093 ) ) 
 REPRESENTATION_ITEM ( '' )  );
#13957=FACE_BOUND ( 'NONE', #267, .T. ) ;
#13960=CARTESIAN_POINT ( 'NONE',  ( 28.56587103547553852, -2.077146556768465047, -5.113484796970851676 ) ) ;
#13961=CARTESIAN_POINT ( 'NONE',  ( 29.36638131047866196, -1.990897739957422807, -5.783357778048658027 ) ) ;
#13974=CARTESIAN_POINT ( 'NONE',  ( 30.37838863598085837, -1.858773980305536089, -5.113484796970855228 ) ) ;
#13977=CARTESIAN_POINT ( 'NONE',  ( 27.30005507882132676, -4.747731375419166788, -3.627061608673664672 ) ) ;
#13980=VECTOR ( 'NONE', #2153, 1000.000000000000114 ) ;
#13981=( BOUNDED_CURVE ( )  B_SPLINE_CURVE ( 2, ( #6783, #10921, #16487, #4160, #13762, #6862, #12393, #12754, #520 ),
 .UNSPECIFIED., .F., .T. ) 
 B_SPLINE_CURVE_WITH_KNOTS ( ( 3, 2, 2, 2, 3 ),
 ( 0.8653846153846154188, 0.8717948717948718063, 0.8846153846153845812, 0.8974358974358974672, 0.9012882778258578531 ),
 .UNSPECIFIED. ) 
 CURVE ( )  GEOMETRIC_REPRESENTATION_ITEM ( )  RATIONAL_B_SPLINE_CURVE ( ( 0.9330127018922192983, 0.9330127018922198534, 1.000000000000000000, 0.8660254037844387076, 1.000000000000000000, 0.8660254037844387076, 1.000000000000000000, 0.9597425536373320742, 0.9436786787937823107 ) ) 
 REPRESENTATION_ITEM ( '' )  );
#13983=EDGE_LOOP ( 'NONE', ( #10877, #6590, #16709, #17556 ) ) ;
#13997=CARTESIAN_POINT ( 'NONE',  ( 30.96820195323705605, -2.125071739898741097, -7.033357778048658027 ) ) ;
#14008=ORIENTED_EDGE ( 'NONE', *, *, #1305, .F. ) ;
#14013=ADVANCED_FACE ( 'NONE', ( #3221, #8763 ), #6016, .T. ) ;
#14019=CARTESIAN_POINT ( 'NONE',  ( 33.58707084003705745, -6.498152266226123963, -5.783357778048669573 ) ) ;
#14026=DIRECTION ( 'NONE',  ( 0.9928203230275512992, 0.1196152422706607682, -0.000000000000000000 ) ) ;
#14029=CARTESIAN_POINT ( 'NONE',  ( 26.01652455409633902, -4.902371455920926380, -5.783357778048663356 ) ) ;
#14035=CARTESIAN_POINT ( 'NONE',  ( 30.52163964716380917, -2.178873678870954400, -4.533357778048659803 ) ) ;
#14040=CARTESIAN_POINT ( 'NONE',  ( 30.04066231269008469, -3.163601260824890904, -7.939653947423660263 ) ) ;
#14043=CARTESIAN_POINT ( 'NONE',  ( 27.14244485254070938, -4.766720295129625029, -7.939653947423662039 ) ) ;
#14047=ORIENTED_EDGE ( 'NONE', *, *, #17557, .F. ) ;
#14051=CARTESIAN_POINT ( 'NONE',  ( 32.22908376348204484, -1.973160382215000785, -7.033357778048658027 ) ) ;
#14052=CARTESIAN_POINT ( 'NONE',  ( 28.97253418081003673, -5.800171738120336151, -7.939653947423664704 ) ) ;
#14058=CARTESIAN_POINT ( 'NONE',  ( 28.12379965168153362, -6.829206799398704675, -7.033357778048666908 ) ) ;
#14067=CARTESIAN_POINT ( 'NONE',  ( 30.44283453230164227, -2.188368138933637574, -4.533357778048659803 ) ) ;
#14069=CARTESIAN_POINT ( 'NONE',  ( 26.46816385032927599, -3.594016774262162262, -3.627061608673662896 ) ) ;
#14075=VERTEX_POINT ( 'NONE', #6648 ) ;
#14079=CARTESIAN_POINT ( 'NONE',  ( 26.31556265977298992, -7.384422263489805793, -5.783357778048663356 ) ) ;
#14080=DIRECTION ( 'NONE',  ( -0.9928203230275512992, -0.1196152422706610180, -4.006172263299093133E-17 ) ) ;
#14081=CARTESIAN_POINT ( 'NONE',  ( 33.13353876934984754, -5.498725377814142945, -8.283357778048662468 ) ) ;
#14103=CARTESIAN_POINT ( 'NONE',  ( 32.97211790677835097, -2.610546234160043610, -8.283357778048660691 ) ) ;
#14113=DIRECTION ( 'NONE',  ( -0.1196152422706599494, 0.9928203230275514102, 0.000000000000000000 ) ) ;
#14121=CARTESIAN_POINT ( 'NONE',  ( 27.95866967485789090, -6.122194908100387245, -3.283357778048667797 ) ) ;
#14125=CARTESIAN_POINT ( 'NONE',  ( 30.67110321781257909, -3.087645581983020637, -7.939653947423660263 ) ) ;
#14127=CARTESIAN_POINT ( 'NONE',  ( 27.24942365487322959, -6.207645047004940686, -3.283357778048667797 ) ) ;
#14130=CONICAL_SURFACE ( 'NONE', #15580, 2.001963570546863025, 0.9599310885968768137 ) ;
#14137=CARTESIAN_POINT ( 'NONE',  ( 33.10345976029034887, -2.594722134608779207, -3.283357778048662023 ) ) ;
#14138=CARTESIAN_POINT ( 'NONE',  ( 33.33308377457396432, -5.274811626130743392, -3.627061608673668225 ) ) ;
#14146=CARTESIAN_POINT ( 'NONE',  ( 30.45719375084302527, -1.849279520242854469, -5.113484796970851676 ) ) ;
#14149=CARTESIAN_POINT ( 'NONE',  ( 31.23537658942770889, -6.791681843624433945, -5.113484796970860558 ) ) ;
#14151=CARTESIAN_POINT ( 'NONE',  ( 26.01652455409633902, -4.902371455920926380, -5.783357778048663356 ) ) ;
#14155=DIRECTION ( 'NONE',  ( 0.1035898384862230515, -0.8598076211353318232, 0.5000000000000001110 ) ) ;
#14161=CARTESIAN_POINT ( 'NONE',  ( 26.01652455409633902, -4.902371455920936150, -5.783357778048664244 ) ) ;
#14170=CARTESIAN_POINT ( 'NONE',  ( 32.57067411085063924, -7.020353038355215070, -5.783357778048669573 ) ) ;
#14176=AXIS2_PLACEMENT_3D ( 'NONE', #3568, #14635, #7289 ) ;
#14193=CARTESIAN_POINT ( 'NONE',  ( 33.56062403295735663, -2.739515387291124426, -3.627061608673662008 ) ) ;
#14202=FACE_OUTER_BOUND ( 'NONE', #2357, .T. ) ;
#14204=ORIENTED_EDGE ( 'NONE', *, *, #15798, .T. ) ;
#14214=CARTESIAN_POINT ( 'NONE',  ( 25.52694003402523748, -4.961356722058193114, -8.283357778048662468 ) ) ;
#14219=CARTESIAN_POINT ( 'NONE',  ( 30.65370992780335868, -5.597623261208691581, -3.627061608673667781 ) ) ;
#14222=CARTESIAN_POINT ( 'NONE',  ( 25.78291734803729796, -2.627872734613073913, -5.430426774474530482 ) ) ;
#14225=EDGE_CURVE ( 'NONE', #17548, #10652, #15443, .T. ) ;
#14226=EDGE_CURVE ( 'NONE', #15670, #13615, #4466, .T. ) ;
#14237=CARTESIAN_POINT ( 'NONE',  ( 33.56515079149260572, -5.873822666371450119, -6.861505862736167138 ) ) ;
#14238=CARTESIAN_POINT ( 'NONE',  ( 30.08145424927873535, -6.930706697444451336, -5.783357778048663356 ) ) ;
#14253=CARTESIAN_POINT ( 'NONE',  ( 27.10313151398701947, -6.652368374500619908, -6.861505862736166250 ) ) ;
#14258=AXIS2_PLACEMENT_3D ( 'NONE', #5407, #16411, #6692 ) ;
#14266=DIRECTION ( 'NONE',  ( 0.1196152422706609902, -0.9928203230275510771, 0.000000000000000000 ) ) ;
#14270=CARTESIAN_POINT ( 'NONE',  ( 30.49166216014303643, -4.363205751385915931, -8.283357778048662468 ) ) ;
#14294=CARTESIAN_POINT ( 'NONE',  ( 33.44685390376565692, -4.007163506710925027, -7.939653947423662039 ) ) ;
#14297=AXIS2_PLACEMENT_3D ( 'NONE', #1546, #8700, #368 ) ;
#14311=LINE ( 'NONE', #7238, #2947 ) ;
#14314=CARTESIAN_POINT ( 'NONE',  ( 26.90793483298706690, -6.248787706170159773, -8.283357778048662468 ) ) ;
#14315=DIRECTION ( 'NONE',  ( -0.9928203230275510771, -0.1196152422706610735, 0.000000000000000000 ) ) ;
#14318=CARTESIAN_POINT ( 'NONE',  ( 30.62726312072365431, -1.838986382273682718, -5.783357778048658027 ) ) ;
#14325=ORIENTED_EDGE ( 'NONE', *, *, #16269, .F. ) ;
#14327=DIRECTION ( 'NONE',  ( 0.9928203230275510771, 0.1196152422706609902, 4.006172263299092517E-17 ) ) ;
#14330=CARTESIAN_POINT ( 'NONE',  ( 28.74176732417158320, -7.092112515190875044, -5.783357778048657138 ) ) ;
#14332=CARTESIAN_POINT ( 'NONE',  ( 25.71072941247523502, -3.058302133056337357, -4.705209693361161349 ) ) ;
#14335=DIRECTION ( 'NONE',  ( -0.05980762113533040492, 0.4964101615137757606, -0.8660254037844384856 ) ) ;
#14338=ORIENTED_EDGE ( 'NONE', *, *, #5837, .T. ) ;
#14345=CARTESIAN_POINT ( 'NONE',  ( 34.23532670761333918, -6.238269840783186027, -9.783357778048662468 ) ) ;
#14347=EDGE_CURVE ( 'NONE', #10379, #16771, #2925, .T. ) ;
#14348=EDGE_CURVE ( 'NONE', #11388, #17192, #3445, .T. ) ;
#14349=CARTESIAN_POINT ( 'NONE',  ( 27.90727577511918867, -2.156494279411373061, -5.783357778048670461 ) ) ;
#14358=CARTESIAN_POINT ( 'NONE',  ( 41.91396146090167463, 0.4627762229654545090, -5.783357778048662468 ) ) ;
#14360=CARTESIAN_POINT ( 'NONE',  ( 32.69820532807177216, -4.097360875439379768, -3.283357778048664688 ) ) ;
#14366=ORIENTED_EDGE ( 'NONE', *, *, #16698, .T. ) ;
#14372=VERTEX_POINT ( 'NONE', #14358 ) ;
#14381=CARTESIAN_POINT ( 'NONE',  ( 32.07220196432897552, -5.426722983814484813, -3.627061608673668225 ) ) ;
#14382=DIRECTION ( 'NONE',  ( -0.9928203230275512992, -0.1196152422706610319, -9.614813431917826478E-17 ) ) ;
#14386=CARTESIAN_POINT ( 'NONE',  ( 26.47269060886452507, -6.728324053342490174, -6.861505862736166250 ) ) ;
#14398=CARTESIAN_POINT ( 'NONE',  ( 25.59340017005574097, -5.757764245108966783, -8.283357778048664244 ) ) ;
#14402=CARTESIAN_POINT ( 'NONE',  ( 26.84461768998868436, -2.294720455324902542, -5.783357778048658027 ) ) ;
#14403=VERTEX_POINT ( 'NONE', #8912 ) ;
#14405=CARTESIAN_POINT ( 'NONE',  ( 26.14833026707293939, -5.996374093462653931, -8.004211544232147091 ) ) ;
#14418=CARTESIAN_POINT ( 'NONE',  ( 32.82963640218302004, -5.962437625020304388, -4.705209693361169343 ) ) ;
#14423=CARTESIAN_POINT ( 'NONE',  ( 28.09001152836988524, -6.106370808549102414, -8.283357778048664244 ) ) ;
#14427=CARTESIAN_POINT ( 'NONE',  ( 31.11087420047036289, -5.742416513891037688, -3.283357778048667797 ) ) ;
#14431=ADVANCED_FACE ( 'NONE', ( #10437 ), #15997, .T. ) ;
#14434=VECTOR ( 'NONE', #6073, 1000.000000000000114 ) ;
#14438=CARTESIAN_POINT ( 'NONE',  ( 31.61111609099199171, -1.710254666422835745, -5.783357778048662468 ) ) ;
#14447=FACE_BOUND ( 'NONE', #7681, .T. ) ;
#14451=CARTESIAN_POINT ( 'NONE',  ( 28.60033944477555323, -4.591072787911525843, -8.283357778048662468 ) ) ;
#14452=CARTESIAN_POINT ( 'NONE',  ( 29.38468146192651886, -6.677295441714964142, -7.033357778048666908 ) ) ;
#14458=CARTESIAN_POINT ( 'NONE',  ( 30.00264913441657555, -6.940201157507134511, -5.783357778048657138 ) ) ;
#14473=CARTESIAN_POINT ( 'NONE',  ( 29.04699097144805364, -6.418171698071525100, -4.705209693361169343 ) ) ;
#14480=CARTESIAN_POINT ( 'NONE',  ( 25.71072941247523502, -3.058302133056337357, -4.705209693361161349 ) ) ;
#14488=CARTESIAN_POINT ( 'NONE',  ( 28.21828588914510050, -7.155181690169023057, -6.453230759126468818 ) ) ;
#14492=CARTESIAN_POINT ( 'NONE',  ( 33.60446413004628141, -3.988174587000466342, -3.627061608673664672 ) ) ;
#14494=PLANE ( 'NONE',  #6071 ) ;
#14495=CARTESIAN_POINT ( 'NONE',  ( 29.51982165028991645, -6.361204938940122844, -4.705209693361168455 ) ) ;
#14499=CARTESIAN_POINT ( 'NONE',  ( 32.33415724766913257, -1.960501102408027219, -4.533357778048659803 ) ) ;
#14512=CARTESIAN_POINT ( 'NONE',  ( 33.56062403295735663, -2.739515387291124426, -3.627061608673662008 ) ) ;
#14514=CARTESIAN_POINT ( 'NONE',  ( 27.58784498402260610, -7.231137369010889770, -6.453230759126474148 ) ) ;
#14516=CARTESIAN_POINT ( 'NONE',  ( 27.46709037723411839, -6.908327297984874882, -4.533357778048668685 ) ) ;
#14524=CARTESIAN_POINT ( 'NONE',  ( 32.67619606237177265, -1.592130426037604352, -5.783357778048658915 ) ) ;
#14527=AXIS2_PLACEMENT_3D ( 'NONE', #8253, #9765, #8522 ) ;
#14533=VECTOR ( 'NONE', #12302, 1000.000000000000114 ) ;
#14538=CARTESIAN_POINT ( 'NONE',  ( 31.63927044622584717, -1.706862622621797110, -5.113484796970854340 ) ) ;
#14541=CARTESIAN_POINT ( 'NONE',  ( 30.00264913441657555, -6.940201157507134511, -5.783357778048657138 ) ) ;
#14543=ORIENTED_EDGE ( 'NONE', *, *, #4199, .T. ) ;
#14545=AXIS2_PLACEMENT_3D ( 'NONE', #13934, #7059, #3663 ) ;
#14550=CARTESIAN_POINT ( 'NONE',  ( 26.66018910156667232, -2.644102211984857842, -4.533357778048659803 ) ) ;
#14564=CARTESIAN_POINT ( 'NONE',  ( 31.86581749455020329, -6.715726164782562790, -5.113484796970860558 ) ) ;
#14574=CARTESIAN_POINT ( 'NONE',  ( 28.93739072872572393, -3.296523698798161650, -7.939653947423660263 ) ) ;
#14579=VECTOR ( 'NONE', #583, 1000.000000000000114 ) ;
#14592=CARTESIAN_POINT ( 'NONE',  ( 27.90727577511918867, -2.156494279411373061, -5.783357778048670461 ) ) ;
#14595=CARTESIAN_POINT ( 'NONE',  ( 31.71314141467879111, -4.216041623526076698, -3.627061608673664672 ) ) ;
#14599=CARTESIAN_POINT ( 'NONE',  ( 28.12741954877813555, -2.767138697495831856, -6.861505862736159145 ) ) ;
#14602=ORIENTED_EDGE ( 'NONE', *, *, #4934, .F. ) ;
#14607=CARTESIAN_POINT ( 'NONE',  ( 29.47916769939009285, -7.003270332485284300, -6.453230759126468818 ) ) ;
#14609=CARTESIAN_POINT ( 'NONE',  ( 29.65098506949083301, -2.583579140294649523, -4.705209693361160461 ) ) ;
#14612=CARTESIAN_POINT ( 'NONE',  ( 32.27410075503257758, -1.240829931302721345, -5.783357778048658027 ) ) ;
#14618=CARTESIAN_POINT ( 'NONE',  ( 32.69811611091622439, -2.216460025892273311, -6.861505862736158257 ) ) ;
#14623=CARTESIAN_POINT ( 'NONE',  ( 32.34851646621051202, -1.621412483717243447, -5.113484796970854340 ) ) ;
#14626=EDGE_CURVE ( 'NONE', #2500, #6811, #5797, .T. ) ;
#14634=CARTESIAN_POINT ( 'NONE',  ( 26.30654288775393113, -7.309557114202778649, -5.423232652803458009 ) ) ;
#14635=DIRECTION ( 'NONE',  ( 0.7020299829125996594, 0.08458074894285609602, -0.7071067811865479058 ) ) ;
#14637=CARTESIAN_POINT ( 'NONE',  ( 28.72045243349238675, -6.030415129707233035, -8.283357778048662468 ) ) ;
#14638=CARTESIAN_POINT ( 'NONE',  ( 30.76748005699505129, -4.329975141788874993, -7.939653947423662039 ) ) ;
#14641=CARTESIAN_POINT ( 'NONE',  ( 29.89119874204131122, -2.254829357712824667, -4.533357778048659803 ) ) ;
#14645=CARTESIAN_POINT ( 'NONE',  ( 31.21213704492286212, -2.822589171134389563, -3.283357778048662023 ) ) ;
#14652=CYLINDRICAL_SURFACE ( 'NONE', #1432, 2.500000000000001776 ) ;
#14654=CARTESIAN_POINT ( 'NONE',  ( 31.41531425212677675, -1.744041783721344219, -5.783357778048658027 ) ) ;
#14659=( BOUNDED_CURVE ( )  B_SPLINE_CURVE ( 2, ( #4995, #11704, #12057, #17561, #7551, #2123, #4810, #11791, #14541 ),
 .UNSPECIFIED., .F., .T. ) 
 B_SPLINE_CURVE_WITH_KNOTS ( ( 3, 2, 2, 2, 3 ),
 ( 0.4807692307692307820, 0.4871794871794871695, 0.5000000000000000000, 0.5128205128205127750, 0.5192307692307692735 ),
 .UNSPECIFIED. ) 
 CURVE ( )  GEOMETRIC_REPRESENTATION_ITEM ( )  RATIONAL_B_SPLINE_CURVE ( ( 0.9330127018922194093, 0.9330127018922196314, 1.000000000000000000, 0.8660254037844387076, 1.000000000000000000, 0.8660254037844387076, 1.000000000000000000, 0.9330127018922187432, 0.9330127018922192983 ) ) 
 REPRESENTATION_ITEM ( '' )  );
#14667=ORIENTED_EDGE ( 'NONE', *, *, #15520, .F. ) ;
#14670=CARTESIAN_POINT ( 'NONE',  ( 27.89480254248674740, -2.495355674045408367, -7.033357778048658027 ) ) ;
#14672=CARTESIAN_POINT ( 'NONE',  ( 32.16857880351144416, -6.669052543620333395, -5.783357778048668685 ) ) ;
#14674=CARTESIAN_POINT ( 'NONE',  ( 31.83134908525019213, -4.201799933639492224, -8.283357778048662468 ) ) ;
#14675=CARTESIAN_POINT ( 'NONE',  ( 27.75549246765397271, -7.200742295513423485, -5.783357778048668685 ) ) ;
#14682=ORIENTED_EDGE ( 'NONE', *, *, #17531, .T. ) ;
#14689=CARTESIAN_POINT ( 'NONE',  ( 29.79859849048667897, -1.928627242885762705, -5.783357778048664244 ) ) ;
#14691=CARTESIAN_POINT ( 'NONE',  ( 28.08810621022444920, -4.652786776866828511, -3.627061608673664672 ) ) ;
#14694=FACE_OUTER_BOUND ( 'NONE', #12894, .T. ) ;
#14700=CARTESIAN_POINT ( 'NONE',  ( 30.91186687973582536, -2.431667782610909434, -4.705209693361160461 ) ) ;
#14704=DIRECTION ( 'NONE',  ( 0.9928203230275512992, 0.1196152422706610735, 9.614813431917828943E-17 ) ) ;
#14707=CARTESIAN_POINT ( 'NONE',  ( 33.20550441965735899, -6.554320347036139971, -5.113484796970860558 ) ) ;
#14712=CARTESIAN_POINT ( 'NONE',  ( 27.92107091181166467, -2.492190854301117753, -4.533357778048659803 ) ) ;
#14722=CARTESIAN_POINT ( 'NONE',  ( 27.42949161418789572, -3.278323244185609830, -3.283357778048662023 ) ) ;
#14724=CARTESIAN_POINT ( 'NONE',  ( 32.14665875496697822, -6.044722943765660439, -6.861505862736166250 ) ) ;
#14732=DIRECTION ( 'NONE',  ( -0.9928203230275512992, -0.1196152422706610180, -4.006172263299093133E-17 ) ) ;
#14739=DIRECTION ( 'NONE',  ( 0.9928203230275510771, 0.1196152422706609902, 4.006172263299092517E-17 ) ) ;
#14741=CARTESIAN_POINT ( 'NONE',  ( 30.80679339554874119, -2.444327062417882779, -6.861505862736158257 ) ) ;
#14743=DIRECTION ( 'NONE',  ( -0.1196152422706606572, 0.9928203230275512992, 0.000000000000000000 ) ) ;
#14744=CARTESIAN_POINT ( 'NONE',  ( 33.23365877489121090, -6.550928303235100891, -5.783357778048663356 ) ) ;
#14747=VERTEX_POINT ( 'NONE', #6897 ) ;
#14752=CARTESIAN_POINT ( 'NONE',  ( 32.87199790123699472, -1.558343308739095656, -5.783357778048663356 ) ) ;
#14753=CIRCLE ( 'NONE', #6344, 3.425051884552432035 ) ;
#14756=ORIENTED_EDGE ( 'NONE', *, *, #15699, .T. ) ;
#14760=CARTESIAN_POINT ( 'NONE',  ( 31.25770402584614516, -1.763030703431812674, -5.783357778048658027 ) ) ;
#14761=DIRECTION ( 'NONE',  ( -0.9928203230275510771, -0.1196152422706614760, -0.000000000000000000 ) ) ;
#14762=CARTESIAN_POINT ( 'NONE',  ( 31.71123609653335507, -2.762457591843783256, -8.283357778048660691 ) ) ;
#14776=LINE ( 'NONE', #11857, #2884 ) ;
#14779=CARTESIAN_POINT ( 'NONE',  ( 29.76058531221316628, -5.705227139567997874, -7.939653947423664704 ) ) ;
#14782=CARTESIAN_POINT ( 'NONE',  ( 31.29094215978502547, -2.813094711071706389, -3.283357778048662023 ) ) ;
#14783=LINE ( 'NONE', #7531, #13374 ) ;
#14784=CARTESIAN_POINT ( 'NONE',  ( 26.87859896403794835, -7.316587507915443211, -6.453230759126474148 ) ) ;
#14787=CARTESIAN_POINT ( 'NONE',  ( 31.55553118839817728, -4.235030543236534939, -7.939653947423662039 ) ) ;
#14792=CARTESIAN_POINT ( 'NONE',  ( 33.23365877489121090, -6.550928303235100891, -5.783357778048663356 ) ) ;
#14808=CARTESIAN_POINT ( 'NONE',  ( 27.18555652250208610, -2.580805812949960920, -7.033357778048658027 ) ) ;
#14809=CARTESIAN_POINT ( 'NONE',  ( 30.90769699326645181, -6.820963901304073929, -5.783357778048668685 ) ) ;
#14822=CARTESIAN_POINT ( 'NONE',  ( 26.01652455409633902, -4.902371455920926380, -5.783357778048663356 ) ) ;
#14825=CARTESIAN_POINT ( 'NONE',  ( 31.04338717100262102, -6.177645381738930297, -6.861505862736167138 ) ) ;
#14827=CARTESIAN_POINT ( 'NONE',  ( 33.27602027394517847, -2.146833986953896822, -4.705209693361161349 ) ) ;
#14857=FACE_OUTER_BOUND ( 'NONE', #8450, .T. ) ;
#14860=CARTESIAN_POINT ( 'NONE',  ( 30.43486631442457835, -6.877930660435475296, -5.783357778048669573 ) ) ;
#14862=ORIENTED_EDGE ( 'NONE', *, *, #7981, .T. ) ;
#14863=CARTESIAN_POINT ( 'NONE',  ( 33.27992013083530054, -6.934902899450660740, -5.783357778048669573 ) ) ;
#14887=CARTESIAN_POINT ( 'NONE',  ( 26.30054492745253825, -7.259773351106304951, -5.235134217867734030 ) ) ;
#14890=CARTESIAN_POINT ( 'NONE',  ( 26.14503574297738098, -5.691300421908874085, -8.283357778048664244 ) ) ;
#14892=CARTESIAN_POINT ( 'NONE',  ( 32.51858583609114106, -1.611119345748072362, -5.783357778048658915 ) ) ;
#14896=ORIENTED_EDGE ( 'NONE', *, *, #6742, .T. ) ;
#14905=CARTESIAN_POINT ( 'NONE',  ( 25.71748644841968456, -2.420320648352046078, -5.783357778048663356 ) ) ;
#14906=CARTESIAN_POINT ( 'NONE',  ( 25.76326615456878244, -3.051972493152843580, -6.861505862736158257 ) ) ;
#14912=ORIENTED_EDGE ( 'NONE', *, *, #11306, .T. ) ;
#14920=EDGE_LOOP ( 'NONE', ( #14325, #12741, #4851 ) ) ;
#14921=CARTESIAN_POINT ( 'NONE',  ( 46.86575133767495061, -2.390451368237048069, -5.783357778048661579 ) ) ;
#14939=DIRECTION ( 'NONE',  ( -0.1196152422706598106, 0.9928203230275514102, 0.000000000000000000 ) ) ;
#14946=CARTESIAN_POINT ( 'NONE',  ( 29.15206445563513071, -6.405512418264540209, -6.861505862736167138 ) ) ;
#14948=CARTESIAN_POINT ( 'NONE',  ( 32.34167700165585302, -2.686501913001913433, -8.283357778048658915 ) ) ;
#14949=CYLINDRICAL_SURFACE ( 'NONE', #17771, 2.500000000000001776 ) ;
#14953=CARTESIAN_POINT ( 'NONE',  ( 27.91310269393460430, -7.181753375802955475, -5.783357778048669573 ) ) ;
#14962=CARTESIAN_POINT ( 'NONE',  ( 28.76992167940542799, -7.088720471389836852, -6.453230759126468818 ) ) ;
#14969=CARTESIAN_POINT ( 'NONE',  ( 26.31376129264122810, -7.369470708288995198, -5.989870097397514748 ) ) ;
#14975=CARTESIAN_POINT ( 'NONE',  ( 32.01513846370018967, -2.298745344637636912, -4.705209693361161349 ) ) ;
#14983=ADVANCED_FACE ( 'NONE', ( #5388 ), #16557, .T. ) ;
#14989=CARTESIAN_POINT ( 'NONE',  ( 33.64386668575551198, -3.983427357176565486, -8.283357778048662468 ) ) ;
#14990=CARTESIAN_POINT ( 'NONE',  ( 25.90899358965569022, -2.397247819800704782, -6.453230759126464378 ) ) ;
#14992=PRODUCT_DEFINITION ( 'UNKNOWN', '', #8028, #5382 ) ;
#14997=DIRECTION ( 'NONE',  ( 0.9928203230275510771, 0.1196152422706609902, 4.006172263299092517E-17 ) ) ;
#15016=VERTEX_POINT ( 'NONE', #6768 ) ;
#15021=CARTESIAN_POINT ( 'NONE',  ( 28.55903157092087952, -3.142235986053133256, -8.283357778048660691 ) ) ;
#15025=CARTESIAN_POINT ( 'NONE',  ( 31.29168529989541270, -6.784897756022354010, -6.453230759126470595 ) ) ;
#15028=CARTESIAN_POINT ( 'NONE',  ( 27.00222791626931595, -2.275731535614434531, -5.783357778048658027 ) ) ;
#15031=CARTESIAN_POINT ( 'NONE',  ( 27.99987602667382802, -2.482696394238434578, -4.533357778048659803 ) ) ;
#15039=CARTESIAN_POINT ( 'NONE',  ( 29.80442540930208750, -6.953886339277345563, -5.783357778048669573 ) ) ;
#15052=CARTESIAN_POINT ( 'NONE',  ( 29.50659824675005893, -4.481886499472614638, -7.939653947423662039 ) ) ;
#15056=CARTESIAN_POINT ( 'NONE',  ( 26.01652455409633902, -4.902371455920926380, -5.783357778048663356 ) ) ;
#15066=CARTESIAN_POINT ( 'NONE',  ( 28.75786045390062995, -2.691183018653962034, -6.861505862736159145 ) ) ;
#15076=( GEOMETRIC_REPRESENTATION_CONTEXT ( 3 ) GLOBAL_UNCERTAINTY_ASSIGNED_CONTEXT ( ( #6809 ) ) GLOBAL_UNIT_ASSIGNED_CONTEXT ( ( #9663, #8057, #12493 ) ) REPRESENTATION_CONTEXT ( 'NONE', 'WORKASPACE' ) );
#15077=VERTEX_POINT ( 'NONE', #11363 ) ;
#15085=CARTESIAN_POINT ( 'NONE',  ( 27.26074174026764751, -6.633379454790151009, -6.861505862736167138 ) ) ;
#15092=VERTEX_POINT ( 'NONE', #3224 ) ;
#15108=ADVANCED_FACE ( 'NONE', ( #1882 ), #16882, .T. ) ;
#15112=ORIENTED_EDGE ( 'NONE', *, *, #5421, .T. ) ;
#15118=DIRECTION ( 'NONE',  ( 0.1196152422706597829, -0.9928203230275514102, 0.000000000000000000 ) ) ;
#15121=CARTESIAN_POINT ( 'NONE',  ( 27.78610916120306129, -6.570083055755264745, -4.705209693361169343 ) ) ;
#15124=CARTESIAN_POINT ( 'NONE',  ( 30.12771560522282499, -7.314681293660012074, -5.783357778048669573 ) ) ;
#15128=( NAMED_UNIT ( * ) PLANE_ANGLE_UNIT ( ) SI_UNIT ( $, .RADIAN. ) );
#15133=CARTESIAN_POINT ( 'NONE',  ( 27.02414796481377124, -2.900061135469103490, -6.861505862736158257 ) ) ;
#15143=( BOUNDED_CURVE ( )  B_SPLINE_CURVE ( 2, ( #11289, #16866, #4514, #14127, #1718, #5867, #11391, #16957, #15577 ),
 .UNSPECIFIED., .F., .T. ) 
 B_SPLINE_CURVE_WITH_KNOTS ( ( 3, 2, 2, 2, 3 ),
 ( 0.8269230769230769829, 0.8333333333333333703, 0.8461538461538461453, 0.8589743589743589203, 0.8653846153846154188 ),
 .UNSPECIFIED. ) 
 CURVE ( )  GEOMETRIC_REPRESENTATION_ITEM ( )  RATIONAL_B_SPLINE_CURVE ( ( 0.9330127018922192983, 0.9330127018922198534, 1.000000000000000000, 0.8660254037844387076, 1.000000000000000000, 0.8660254037844387076, 1.000000000000000000, 0.9330127018922187432, 0.9330127018922192983 ) ) 
 REPRESENTATION_ITEM ( '' )  );
#15144=CARTESIAN_POINT ( 'NONE',  ( 33.68284756902015431, -1.652629194728084450, -1.783357778048662912 ) ) ;
#15145=DIRECTION ( 'NONE',  ( 0.9928203230275510771, 0.1196152422706609902, 4.006172263299092517E-17 ) ) ;
#15146=CARTESIAN_POINT ( 'NONE',  ( 29.49337484321020497, -2.602568060005117090, -4.705209693361161349 ) ) ;
#15156=CARTESIAN_POINT ( 'NONE',  ( 26.31556265977298992, -7.384422263489805793, -5.783357778048663356 ) ) ;
#15159=CARTESIAN_POINT ( 'NONE',  ( 25.92467471225709374, -2.732717170633701453, -7.033357778048658027 ) ) ;
#15160=CARTESIAN_POINT ( 'NONE',  ( 27.72904566057427189, -3.442105416578421284, -3.627061608673662896 ) ) ;
#15163=CARTESIAN_POINT ( 'NONE',  ( 32.60321786976872005, -6.626883982076972934, -5.783357778048663356 ) ) ;
#15176=CARTESIAN_POINT ( 'NONE',  ( 28.28955653359400557, -5.882457056865704637, -3.627061608673668225 ) ) ;
#15186=CARTESIAN_POINT ( 'NONE',  ( 26.01652455409633902, -4.902371455920926380, -5.783357778048663356 ) ) ;
#15208=CARTESIAN_POINT ( 'NONE',  ( 27.23882169172318513, -6.009049854935478052, -7.939653947423664704 ) ) ;
#15209=CARTESIAN_POINT ( 'NONE',  ( 28.76917853929504432, -3.116917426439186123, -3.283357778048662023 ) ) ;
#15214=ORIENTED_EDGE ( 'NONE', *, *, #6280, .F. ) ;
#15216=CARTESIAN_POINT ( 'NONE',  ( 28.71854711534694715, -4.576831098024959132, -3.627061608673664672 ) ) ;
#15220=EDGE_LOOP ( 'NONE', ( #4710, #11741, #12280, #4350 ) ) ;
#15229=CARTESIAN_POINT ( 'NONE',  ( 29.45101334415624095, -7.006662376286321603, -5.783357778048657138 ) ) ;
#15230=CARTESIAN_POINT ( 'NONE',  ( 30.15026255541241440, -6.285249260098253465, -4.705209693361168455 ) ) ;
#15232=CYLINDRICAL_SURFACE ( 'NONE', #1476, 2.500000000000001776 ) ;
#15240=CARTESIAN_POINT ( 'NONE',  ( 27.50150540219088313, -5.977401655418041138, -3.627061608673667781 ) ) ;
#15250=( BOUNDED_CURVE ( )  B_SPLINE_CURVE ( 2, ( #15568, #9933, #3065, #12581, #161 ),
 .UNSPECIFIED., .F., .F. ) 
 B_SPLINE_CURVE_WITH_KNOTS ( ( 3, 2, 3 ),
 ( 0.000000000000000000, 0.01282051282051282007, 0.01923076923076924918 ),
 .UNSPECIFIED. ) 
 CURVE ( )  GEOMETRIC_REPRESENTATION_ITEM ( )  RATIONAL_B_SPLINE_CURVE ( ( 1.000000000000000000, 0.8660254037844387076, 1.000000000000000000, 0.9330127018922191873, 0.9330127018922194093 ) ) 
 REPRESENTATION_ITEM ( '' )  );
#15251=EDGE_CURVE ( 'NONE', #8853, #13220, #5845, .T. ) ;
#15256=CARTESIAN_POINT ( 'NONE',  ( 25.99533317148741318, -3.650983533393564517, -3.627061608673662008 ) ) ;
#15260=SURFACE_STYLE_USAGE ( .BOTH. , #1177 ) ;
#15265=( NAMED_UNIT ( * ) SI_UNIT ( $, .STERADIAN. ) SOLID_ANGLE_UNIT ( ) );
#15273=CARTESIAN_POINT ( 'NONE',  ( 28.82057243903374655, -7.082618055128190093, -5.783357778048668685 ) ) ;
#15277=CIRCLE ( 'NONE', #7469, 2.001963570546864801 ) ;
#15291=DIRECTION ( 'NONE',  ( -0.1196152422706610735, 0.9928203230275511881, 0.000000000000000000 ) ) ;
#15295=CARTESIAN_POINT ( 'NONE',  ( 26.19678349485696955, -4.880653813392439311, -3.627061608673664672 ) ) ;
#15296=CARTESIAN_POINT ( 'NONE',  ( 26.28630169594996246, -7.141552884944044166, -6.905585309297165963 ) ) ;
#15297=CARTESIAN_POINT ( 'NONE',  ( 30.48043329534786849, -5.818372192732907067, -3.283357778048667797 ) ) ;
#15298=CARTESIAN_POINT ( 'NONE',  ( 32.52441275490655670, -6.636378442139655220, -5.783357778048663356 ) ) ;
#15302=CARTESIAN_POINT ( 'NONE',  ( 31.51621784984448738, -6.120678622607529817, -6.861505862736166250 ) ) ;
#15305=CARTESIAN_POINT ( 'NONE',  ( 28.49970350196817392, -5.857138497251737519, -7.939653947423662927 ) ) ;
#15317=CARTESIAN_POINT ( 'NONE',  ( 30.45225960443380231, -4.367952981209816343, -3.627061608673664672 ) ) ;
#15327=CARTESIAN_POINT ( 'NONE',  ( 33.60446413004628141, -3.988174587000466342, -3.627061608673664672 ) ) ;
#15331=CARTESIAN_POINT ( 'NONE',  ( 28.34209327568754944, -5.876127416962207306, -7.939653947423662927 ) ) ;
#15339=ORIENTED_EDGE ( 'NONE', *, *, #12198, .T. ) ;
#15340=VECTOR ( 'NONE', #9936, 1000.000000000000227 ) ;
#15349=CARTESIAN_POINT ( 'NONE',  ( 32.38298487551052318, -4.135338714860305132, -8.283357778048662468 ) ) ;
#15371=CARTESIAN_POINT ( 'NONE',  ( 31.87075164095941915, -4.197052703815608687, -3.627061608673664672 ) ) ;
#15376=VERTEX_POINT ( 'NONE', #9197 ) ;
#15378=EDGE_CURVE ( 'NONE', #15077, #12431, #2961, .T. ) ;
#15381=CARTESIAN_POINT ( 'NONE',  ( 31.51612863268893960, -4.239777773060436239, -3.283357778048664688 ) ) ;
#15387=DIRECTION ( 'NONE',  ( 0.9928203230275512992, 0.1196152422706610180, 4.006172263299093133E-17 ) ) ;
#15391=EDGE_CURVE ( 'NONE', #16897, #17484, #13195, .T. ) ;
#15392=CARTESIAN_POINT ( 'NONE',  ( 30.72436838703367812, -6.515889623968540434, -7.033357778048666908 ) ) ;
#15397=CARTESIAN_POINT ( 'NONE',  ( 30.12381574833269937, -2.526612381163247267, -4.705209693361161349 ) ) ;
#15398=ORIENTED_EDGE ( 'NONE', *, *, #1087, .T. ) ;
#15400=CARTESIAN_POINT ( 'NONE',  ( 26.82722439997946395, -4.804698134550569044, -3.627061608673664672 ) ) ;
#15406=VERTEX_POINT ( 'NONE', #15828 ) ;
#15411=CARTESIAN_POINT ( 'NONE',  ( 32.24155699611449677, -1.634298987580965923, -5.783357778048664244 ) ) ;
#15412=CARTESIAN_POINT ( 'NONE',  ( 33.75714020991769360, -6.487859128256953767, -5.113484796970860558 ) ) ;
#15413=CARTESIAN_POINT ( 'NONE',  ( 29.19137779418881351, -4.519864338893556877, -3.627061608673664672 ) ) ;
#15416=AXIS2_PLACEMENT_3D ( 'NONE', #7672, #14382, #14743 ) ;
#15428=CARTESIAN_POINT ( 'NONE',  ( 28.98992747081926069, -3.290194058894681639, -3.627061608673662896 ) ) ;
#15431=EDGE_CURVE ( 'NONE', #2990, #17907, #6212, .T. ) ;
#15439=AXIS2_PLACEMENT_3D ( 'NONE', #7190, #3016, #2913 ) ;
#15443=LINE ( 'NONE', #9622, #16792 ) ;
#15445=CARTESIAN_POINT ( 'NONE',  ( 31.56485473504790917, -1.326280070207274564, -5.783357778048658027 ) ) ;
#15453=SURFACE_SIDE_STYLE ('',( #3036 ) ) ;
#15465=CARTESIAN_POINT ( 'NONE',  ( 32.69811611091622439, -2.216460025892273311, -6.861505862736158257 ) ) ;
#15466=ADVANCED_FACE ( 'NONE', ( #13281 ), #2849, .T. ) ;
#15474=CARTESIAN_POINT ( 'NONE',  ( 31.05948030073166066, -1.776715885202022394, -5.783357778048662468 ) ) ;
#15485=CARTESIAN_POINT ( 'NONE',  ( 33.27602027394517847, -2.146833986953896822, -4.705209693361161349 ) ) ;
#15488=CARTESIAN_POINT ( 'NONE',  ( 31.71314141467879111, -4.216041623526076698, -3.627061608673664672 ) ) ;
#15491=CARTESIAN_POINT ( 'NONE',  ( 25.80383423833348644, -3.137017275366889901, -7.141595990038014818 ) ) ;
#15502=CARTESIAN_POINT ( 'NONE',  ( 33.32864623319426300, -4.021405196597508613, -3.283357778048664688 ) ) ;
#15503=CARTESIAN_POINT ( 'NONE',  ( 31.69574812466957781, -6.726019302751734763, -5.783357778048669573 ) ) ;
#15516=CARTESIAN_POINT ( 'NONE',  ( 26.03917326857634151, -4.899642733102906433, -3.627061608673664672 ) ) ;
#15517=ORIENTED_EDGE ( 'NONE', *, *, #11765, .T. ) ;
#15520=EDGE_CURVE ( 'NONE', #14075, #4809, #13981, .T. ) ;
#15524=ORIENTED_EDGE ( 'NONE', *, *, #875, .T. ) ;
#15529=CARTESIAN_POINT ( 'NONE',  ( 32.82573654529290508, -1.174368712523534475, -5.783357778048658027 ) ) ;
#15556=CARTESIAN_POINT ( 'NONE',  ( 25.77727942049545717, -5.625018267156629115, -7.939653947423662039 ) ) ;
#15558=EDGE_CURVE ( 'NONE', #7189, #8269, #14311, .T. ) ;
#15561=DIRECTION ( 'NONE',  ( -0.1196152422706610735, 0.9928203230275511881, 0.000000000000000000 ) ) ;
#15562=ORIENTED_EDGE ( 'NONE', *, *, #1087, .F. ) ;
#15566=CARTESIAN_POINT ( 'NONE',  ( 31.89397184978405519, -6.712334120981523711, -5.783357778048663356 ) ) ;
#15567=FACE_OUTER_BOUND ( 'NONE', #9888, .T. ) ;
#15568=CARTESIAN_POINT ( 'NONE',  ( 33.95908713831676096, -3.945449517755638791, -3.283357778048664688 ) ) ;
#15570=CARTESIAN_POINT ( 'NONE',  ( 26.06734695949040059, -6.350061944625998933, -3.283357778048667797 ) ) ;
#15575=CARTESIAN_POINT ( 'NONE',  ( 32.14665875496697822, -6.044722943765660439, -6.861505862736166250 ) ) ;
#15576=CARTESIAN_POINT ( 'NONE',  ( 27.02867472334902033, -6.034368414549445170, -3.627061608673668225 ) ) ;
#15577=CARTESIAN_POINT ( 'NONE',  ( 26.56758885001203652, -2.317900097157796324, -5.783357778048670461 ) ) ;
#15578=ORIENTED_EDGE ( 'NONE', *, *, #5265, .F. ) ;
#15580=AXIS2_PLACEMENT_3D ( 'NONE', #12772, #1725, #8422 ) ;
#15581=ORIENTED_EDGE ( 'NONE', *, *, #9618, .F. ) ;
#15584=FACE_OUTER_BOUND ( 'NONE', #8732, .T. ) ;
#15589=CARTESIAN_POINT ( 'NONE',  ( 33.58707084003705745, -6.498152266226123963, -5.783357778048669573 ) ) ;
#15591=CARTESIAN_POINT ( 'NONE',  ( 27.53837573810955419, -6.172832027328289506, -8.283357778048664244 ) ) ;
#15592=AXIS2_PLACEMENT_3D ( 'NONE', #7912, #13447, #1028 ) ;
#15621=CARTESIAN_POINT ( 'NONE',  ( 32.53688598753899441, -6.297517047505613697, -7.033357778048666908 ) ) ;
#15625=VERTEX_POINT ( 'NONE', #17132 ) ;
#15629=CARTESIAN_POINT ( 'NONE',  ( 30.42903939560917337, -1.852671564043892660, -5.783357778048658027 ) ) ;
#15633=CARTESIAN_POINT ( 'NONE',  ( 26.31556265977298992, -7.384422263489805793, -5.783357778048663356 ) ) ;
#15637=CARTESIAN_POINT ( 'NONE',  ( 26.39379627684682106, -4.856917663858078882, -3.283357778048664688 ) ) ;
#15639=FACE_OUTER_BOUND ( 'NONE', #16109, .T. ) ;
#15645=CARTESIAN_POINT ( 'NONE',  ( 32.06767520579373354, -2.292415704734142690, -6.861505862736158257 ) ) ;
#15653=ADVANCED_FACE ( 'NONE', ( #15567 ), #252, .F. ) ;
#15664=CARTESIAN_POINT ( 'NONE',  ( 26.03726795043090547, -3.446058701420613879, -8.283357778048658915 ) ) ;
#15669=CARTESIAN_POINT ( 'NONE',  ( 31.53813789838894621, -6.745008222462202774, -5.783357778048668685 ) ) ;
#15670=VERTEX_POINT ( 'NONE', #11277 ) ;
#15684=CARTESIAN_POINT ( 'NONE',  ( 30.91186687973582536, -2.431667782610909434, -4.705209693361160461 ) ) ;
#15686=CARTESIAN_POINT ( 'NONE',  ( 27.27683486999669427, -2.232449958253242883, -5.783357778048658027 ) ) ;
#15689=CARTESIAN_POINT ( 'NONE',  ( 28.09753128235661279, -6.832371619143005503, -4.533357778048668685 ) ) ;
#15699=EDGE_CURVE ( 'NONE', #317, #16897, #7597, .T. ) ;
#15701=CARTESIAN_POINT ( 'NONE',  ( 26.45077056032005913, -6.103994453487816330, -7.939653947423662927 ) ) ;
#15705=CYLINDRICAL_SURFACE ( 'NONE', #15439, 2.500000000000001776 ) ;
#15720=CARTESIAN_POINT ( 'NONE',  ( 28.45891156537951971, -2.090033060632186412, -5.783357778048670461 ) ) ;
#15723=CARTESIAN_POINT ( 'NONE',  ( 30.17644170758179101, -4.401183590806859947, -3.283357778048664688 ) ) ;
#15725=CARTESIAN_POINT ( 'NONE',  ( 29.23078034989804763, -4.515117109069654688, -8.283357778048662468 ) ) ;
#15728=CARTESIAN_POINT ( 'NONE',  ( 30.69058026372202974, -5.793053633118939061, -8.283357778048664244 ) ) ;
#15729=CARTESIAN_POINT ( 'NONE',  ( 29.82675284572052732, -1.925235199084722959, -5.113484796970855228 ) ) ;
#15737=DIRECTION ( 'NONE',  ( -0.05980762113533042573, 0.4964101615137759271, -0.8660254037844383745 ) ) ;
#15743=EDGE_CURVE ( 'NONE', #16997, #627, #6559, .T. ) ;
#15749=CARTESIAN_POINT ( 'NONE',  ( 33.68284756902015431, -1.652629194728085338, -9.783357778048662468 ) ) ;
#15756=CARTESIAN_POINT ( 'NONE',  ( 26.01652455409633902, -4.902371455920926380, -5.783357778048663356 ) ) ;
#15761=CARTESIAN_POINT ( 'NONE',  ( 26.87785582392756467, -3.344784462964796479, -3.283357778048662023 ) ) ;
#15765=CARTESIAN_POINT ( 'NONE',  ( 28.77978050244509944, -3.315512618508630993, -7.939653947423660263 ) ) ;
#15766=CARTESIAN_POINT ( 'NONE',  ( 25.79194807336802953, -3.038360733637177624, -6.974889548725401234 ) ) ;
#15769=VERTEX_POINT ( 'NONE', #17515 ) ;
#15777=CARTESIAN_POINT ( 'NONE',  ( 25.60565592828815440, -3.070961412863312034, -6.861505862736159145 ) ) ;
#15781=CARTESIAN_POINT ( 'NONE',  ( 26.67454832010805532, -2.305013593294074514, -5.113484796970851676 ) ) ;
#15796=FACE_OUTER_BOUND ( 'NONE', #13906, .T. ) ;
#15797=CARTESIAN_POINT ( 'NONE',  ( 33.48996557372703364, -1.821249024531260696, -7.033357778048658027 ) ) ;
#15798=EDGE_CURVE ( 'NONE', #4809, #15874, #16137, .T. ) ;
#15801=CARTESIAN_POINT ( 'NONE',  ( 26.55511561737958814, -2.656761491791831187, -7.033357778048658027 ) ) ;
#15804=CARTESIAN_POINT ( 'NONE',  ( 26.01652455409633902, -4.902371455920926380, -5.783357778048663356 ) ) ;
#15807=CARTESIAN_POINT ( 'NONE',  ( 27.45957062324739795, -6.182326487390973568, -8.283357778048662468 ) ) ;
#15816=DIRECTION ( 'NONE',  ( 0.9928203230275512992, 0.1196152422706587698, 0.000000000000000000 ) ) ;
#15818=EDGE_CURVE ( 'NONE', #12534, #692, #5205, .T. ) ;
#15819=CARTESIAN_POINT ( 'NONE',  ( 26.75784435724945709, -6.993777436889428323, -4.533357778048668685 ) ) ;
#15820=DIRECTION ( 'NONE',  ( -0.6047431568147647596, -0.4535573676110720709, 0.6546536707079764206 ) ) ;
#15827=CARTESIAN_POINT ( 'NONE',  ( 30.30787278169304244, -6.266260340387784566, -4.705209693361169343 ) ) ;
#15828=CARTESIAN_POINT ( 'NONE',  ( 42.73333828282231650, -6.338146013849483396, -5.783357778048662468 ) ) ;
#15833=CARTESIAN_POINT ( 'NONE',  ( 26.25801688195511474, -3.619335333876111171, -7.939653947423660263 ) ) ;
#15842=ADVANCED_FACE ( 'NONE', ( #7767 ), #13296, .T. ) ;
#15845=CARTESIAN_POINT ( 'NONE',  ( 25.40682704530840397, -3.522014380262483702, -8.283357778048658915 ) ) ;
#15849=CARTESIAN_POINT ( 'NONE',  ( 27.71165237056504438, -5.952083095804076684, -7.939653947423664704 ) ) ;
#15867=CARTESIAN_POINT ( 'NONE',  ( 32.18597209352066812, -4.159074864394664672, -7.939653947423662039 ) ) ;
#15874=VERTEX_POINT ( 'NONE', #11079 ) ;
#15876=CARTESIAN_POINT ( 'NONE',  ( 32.95662993491456660, -6.574107945067995118, -5.783357778048669573 ) ) ;
#15887=CARTESIAN_POINT ( 'NONE',  ( 29.77118727536321074, -5.903822331637461396, -3.283357778048667797 ) ) ;
#15888=DIRECTION ( 'NONE',  ( 0.6047431568147660919, 0.4535573676110685737, 0.6546536707079775308 ) ) ;
#15898=CARTESIAN_POINT ( 'NONE',  ( 27.02423718196931546, -4.780961985016209503, -3.283357778048664688 ) ) ;
#15905=CARTESIAN_POINT ( 'NONE',  ( 30.68374079916737429, -6.858143062403621926, -5.113484796970860558 ) ) ;
#15907=ORIENTED_EDGE ( 'NONE', *, *, #7022, .T. ) ;
#15910=CARTESIAN_POINT ( 'NONE',  ( 25.85239768453567066, -3.540099486550932983, -4.114102314938801186 ) ) ;
#15914=VECTOR ( 'NONE', #1167, 1000.000000000000227 ) ;
#15918=CARTESIAN_POINT ( 'NONE',  ( 31.67382807612511542, -6.101689702897060030, -6.861505862736167138 ) ) ;
#15926=VERTEX_POINT ( 'NONE', #12195 ) ;
#15927=AXIS2_PLACEMENT_3D ( 'NONE', #14921, #10894, #9463 ) ;
#15928=CARTESIAN_POINT ( 'NONE',  ( 25.60565592828815440, -3.070961412863312034, -6.861505862736159145 ) ) ;
#15932=CARTESIAN_POINT ( 'NONE',  ( 27.33945763453056088, -4.742984145595265488, -8.283357778048662468 ) ) ;
#15934=ORIENTED_EDGE ( 'NONE', *, *, #2656, .F. ) ;
#15940=CARTESIAN_POINT ( 'NONE',  ( 31.51169109130924184, -2.986371343527201905, -3.627061608673662896 ) ) ;
#15942=DIRECTION ( 'NONE',  ( -0.1035898384862230376, 0.8598076211353316012, 0.5000000000000004441 ) ) ;
#15944=CARTESIAN_POINT ( 'NONE',  ( 28.13194630731337753, -5.901445976576171759, -3.627061608673667781 ) ) ;
#15951=ORIENTED_EDGE ( 'NONE', *, *, #14226, .F. ) ;
#15961=STYLED_ITEM ( 'NONE', ( #2530 ), #7664 ) ;
#15963=CARTESIAN_POINT ( 'NONE',  ( 30.40841950734487753, -3.119293781500474427, -3.627061608673662008 ) ) ;
#15967=CARTESIAN_POINT ( 'NONE',  ( 31.04700706809921940, -2.115577279836057922, -7.033357778048658027 ) ) ;
#15971=ORIENTED_EDGE ( 'NONE', *, *, #6043, .F. ) ;
#15972=VECTOR ( 'NONE', #9333, 1000.000000000000114 ) ;
#15973=ORIENTED_EDGE ( 'NONE', *, *, #6986, .T. ) ;
#15975=B_SPLINE_CURVE_WITH_KNOTS ( 'NONE', 3,
 ( #3890, #1170, #6690, #8146, #17203, #15296, #10086, #4746 ),
 .UNSPECIFIED., .F., .F.,
 ( 4, 2, 2, 4 ),
 ( 0.8481424625553403152, 0.8776269672338687933, 0.9071114719123971604, 0.9660804812694540056 ),
 .UNSPECIFIED. ) ;
#15976=CARTESIAN_POINT ( 'NONE',  ( 31.67382807612511542, -6.101689702897060030, -6.861505862736167138 ) ) ;
#15979=VECTOR ( 'NONE', #2898, 999.9999999999998863 ) ;
#15997=PLANE ( 'NONE',  #14176 ) ;
#15999=CARTESIAN_POINT ( 'NONE',  ( 27.29063000668916672, -2.568146533142987575, -4.533357778048659803 ) ) ;
#16000=CARTESIAN_POINT ( 'NONE',  ( 30.75425665345519732, -2.450656702321377001, -4.705209693361161349 ) ) ;
#16009=CARTESIAN_POINT ( 'NONE',  ( 25.76524775868381667, -2.816745038626284892, -5.277258820486252944 ) ) ;
#16019=CYLINDRICAL_SURFACE ( 'NONE', #6570, 2.500000000000001776 ) ;
#16022=CARTESIAN_POINT ( 'NONE',  ( 28.91999743871649997, -5.806501378023834370, -3.627061608673668225 ) ) ;
#16030=EDGE_LOOP ( 'NONE', ( #4217, #6684, #6680, #564 ) ) ;
#16042=CARTESIAN_POINT ( 'NONE',  ( 31.51621784984448738, -6.120678622607529817, -6.861505862736166250 ) ) ;
#16046=CARTESIAN_POINT ( 'NONE',  ( 29.01637427789896151, -7.048830937829683840, -5.783357778048668685 ) ) ;
#16054=LINE ( 'NONE', #3623, #12664 ) ;
#16058=CARTESIAN_POINT ( 'NONE',  ( 29.15568435273173264, -2.343444316361667834, -7.033357778048658027 ) ) ;
#16060=CARTESIAN_POINT ( 'NONE',  ( 28.30694982360322953, -3.372479377640031473, -7.939653947423660263 ) ) ;
#16061=CARTESIAN_POINT ( 'NONE',  ( 30.66124439477291475, -6.860853434864224276, -6.453230759126470595 ) ) ;
#16063=CARTESIAN_POINT ( 'NONE',  ( 32.90454166015506132, -1.164874252460851300, -5.783357778048658027 ) ) ;
#16070=CARTESIAN_POINT ( 'NONE',  ( 32.32618902979206865, -6.650063623909865385, -5.783357778048669573 ) ) ;
#16082=ADVANCED_FACE ( 'NONE', ( #15639 ), #11538, .T. ) ;
#16090=CARTESIAN_POINT ( 'NONE',  ( 28.28511899221430070, -4.629050627332469858, -3.283357778048664688 ) ) ;
#16091=CARTESIAN_POINT ( 'NONE',  ( 32.56242593318006584, -2.859778545457409837, -7.939653947423660263 ) ) ;
#16092=EDGE_CURVE ( 'NONE', #15670, #16642, #17831, .T. ) ;
#16093=EDGE_LOOP ( 'NONE', ( #5896, #5082, #8960, #4409 ) ) ;
#16099=EDGE_LOOP ( 'NONE', ( #11328, #5167, #15214, #13050 ) ) ;
#16109=EDGE_LOOP ( 'NONE', ( #7874, #14047, #4709, #10171 ) ) ;
#16110=CARTESIAN_POINT ( 'NONE',  ( 29.02054416436834217, -2.659534819136519790, -4.705209693361160461 ) ) ;
#16111=CARTESIAN_POINT ( 'NONE',  ( 33.40660799972355477, 0.6401911282994665608, -5.783357778048661579 ) ) ;
#16115=EDGE_CURVE ( 'NONE', #8269, #3859, #1874, .T. ) ;
#16123=DIRECTION ( 'NONE',  ( 0.000000000000000000, 0.5027044994213119011, 0.8644583195629320649 ) ) ;
#16125=CARTESIAN_POINT ( 'NONE',  ( 26.31556265977298992, -7.384422263489805793, -5.783357778048663356 ) ) ;
#16127=CARTESIAN_POINT ( 'NONE',  ( 32.79901970863393501, -6.593096864778464017, -5.783357778048668685 ) ) ;
#16130=CARTESIAN_POINT ( 'NONE',  ( 28.97253418081003673, -5.800171738120336151, -7.939653947423664704 ) ) ;
#16137=B_SPLINE_CURVE_WITH_KNOTS ( 'NONE', 3,
 ( #13481, #6226, #8948, #17414, #17685 ),
 .UNSPECIFIED., .F., .F.,
 ( 4, 1, 4 ),
 ( 0.9660804812694540056, 0.9703207337145166589, 0.9745609861595793122 ),
 .UNSPECIFIED. ) ;
#16146=CARTESIAN_POINT ( 'NONE',  ( 30.60986983071443390, -4.348964061499348333, -3.627061608673664672 ) ) ;
#16148=CARTESIAN_POINT ( 'NONE',  ( 31.88017671309158274, -6.376637546091784792, -4.533357778048668685 ) ) ;
#16154=CARTESIAN_POINT ( 'NONE',  ( 32.06767520579373354, -2.292415704734142690, -6.861505862736158257 ) ) ;
#16173=CARTESIAN_POINT ( 'NONE',  ( 25.97837335112617652, -4.585712065882579402, -3.626324104489874411 ) ) ;
#16176=CARTESIAN_POINT ( 'NONE',  ( 29.14074637024071635, -5.979778010479330774, -3.283357778048667797 ) ) ;
#16177=CARTESIAN_POINT ( 'NONE',  ( 32.16857880351144416, -6.669052543620333395, -5.783357778048668685 ) ) ;
#16194=CARTESIAN_POINT ( 'NONE',  ( 26.01652455409633902, -4.902371455920926380, -5.783357778048663356 ) ) ;
#16197=CARTESIAN_POINT ( 'NONE',  ( 30.92509028327567933, -4.310986222078405206, -7.939653947423662039 ) ) ;
#16198=AXIS2_PLACEMENT_3D ( 'NONE', #12032, #17794, #15118 ) ;
#16199=CARTESIAN_POINT ( 'NONE',  ( 33.38562051666750818, -5.268481986227246061, -7.939653947423664704 ) ) ;
#16204=AXIS2_PLACEMENT_3D ( 'NONE', #6115, #11643, #17210 ) ;
#16209=VECTOR ( 'NONE', #8283, 1000.000000000000000 ) ;
#16232=CARTESIAN_POINT ( 'NONE',  ( 29.34898802046944155, -4.500875419183088866, -3.627061608673664672 ) ) ;
#16235=CARTESIAN_POINT ( 'NONE',  ( 33.40745134805642635, -4.011910736534825439, -3.283357778048664688 ) ) ;
#16244=CARTESIAN_POINT ( 'NONE',  ( 30.40841950734487753, -3.119293781500474427, -3.627061608673662008 ) ) ;
#16252=VECTOR ( 'NONE', #6708, 1000.000000000000114 ) ;
#16253=LINE ( 'NONE', #5428, #4962 ) ;
#16267=CARTESIAN_POINT ( 'NONE',  ( 33.42946061375642586, -6.517141185936593750, -5.783357778048668685 ) ) ;
#16269=EDGE_CURVE ( 'NONE', #15926, #14747, #11064, .T. ) ;
#16282=DIRECTION ( 'NONE',  ( 0.9928203230275510771, 0.1196152422706609902, 4.006172263299092517E-17 ) ) ;
#16285=CARTESIAN_POINT ( 'NONE',  ( 26.05393439953038381, -7.587479618990243146, -6.529799540429926274 ) ) ;
#16297=FACE_OUTER_BOUND ( 'NONE', #2801, .T. ) ;
#16315=VERTEX_POINT ( 'NONE', #852 ) ;
#16317=ADVANCED_FACE ( 'NONE', ( #13271 ), #2407, .F. ) ;
#16322=VERTEX_POINT ( 'NONE', #1039 ) ;
#16325=AXIS2_PLACEMENT_3D ( 'NONE', #12269, #14732, #7924 ) ;
#16327=CARTESIAN_POINT ( 'NONE',  ( 28.89355063163679915, -2.047864499088824175, -5.783357778048658027 ) ) ;
#16330=CARTESIAN_POINT ( 'NONE',  ( 33.21234388421201089, -5.489230917751459771, -8.283357778048662468 ) ) ;
#16331=FACE_OUTER_BOUND ( 'NONE', #5592, .T. ) ;
#16338=CARTESIAN_POINT ( 'NONE',  ( 30.15443244188179150, -1.895953141405083864, -5.783357778048658915 ) ) ;
#16346=EDGE_CURVE ( 'NONE', #5903, #13433, #4747, .T. ) ;
#16350=CARTESIAN_POINT ( 'NONE',  ( 28.44643833274707845, -2.428894455266221275, -7.033357778048658027 ) ) ;
#16360=CARTESIAN_POINT ( 'NONE',  ( 26.39379627684682106, -4.856917663858078882, -3.283357778048664688 ) ) ;
#16361=CARTESIAN_POINT ( 'NONE',  ( 33.19286683830256379, -2.783822866615540459, -7.939653947423660263 ) ) ;
#16374=CARTESIAN_POINT ( 'NONE',  ( 25.74134610602432360, -2.427642893298174620, -5.783357778048658027 ) ) ;
#16396=ORIENTED_EDGE ( 'NONE', *, *, #3693, .T. ) ;
#16411=DIRECTION ( 'NONE',  ( 0.9928203230275512992, 0.1196152422706610180, 4.006172263299093133E-17 ) ) ;
#16417=CARTESIAN_POINT ( 'NONE',  ( 29.13014440709066832, -5.781182818409868140, -7.939653947423662927 ) ) ;
#16421=EDGE_LOOP ( 'NONE', ( #11802, #10289, #1068, #9730 ) ) ;
#16425=CARTESIAN_POINT ( 'NONE',  ( 32.26287188679368256, -2.695996373064596607, -8.283357778048660691 ) ) ;
#16427=CARTESIAN_POINT ( 'NONE',  ( 28.56093688906631911, -4.595820017735426255, -3.627061608673664672 ) ) ;
#16439=CARTESIAN_POINT ( 'NONE',  ( 30.27725608814395386, -6.896919580145944195, -5.783357778048668685 ) ) ;
#16454=CARTESIAN_POINT ( 'NONE',  ( 25.86833963875586306, -3.039313213345869791, -4.705209693361160461 ) ) ;
#16464=LINE ( 'NONE', #16546, #1450 ) ;
#16467=LINE ( 'NONE', #5297, #8645 ) ;
#16473=CARTESIAN_POINT ( 'NONE',  ( 26.01652455409633902, -4.902371455920926380, -5.783357778048663356 ) ) ;
#16487=CARTESIAN_POINT ( 'NONE',  ( 26.00347982711925710, -2.723222710571018279, -7.033357778048658027 ) ) ;
#16489=CARTESIAN_POINT ( 'NONE',  ( 31.38859741546781379, -7.162769935976271540, -5.783357778048669573 ) ) ;
#16491=CARTESIAN_POINT ( 'NONE',  ( 42.32364987186199556, -2.937684895442014277, -5.783357778048662468 ) ) ;
#16496=CARTESIAN_POINT ( 'NONE',  ( 29.56783163384821833, -3.220568019956291383, -7.939653947423660263 ) ) ;
#16501=ORIENTED_EDGE ( 'NONE', *, *, #15818, .T. ) ;
#16502=( BOUNDED_CURVE ( )  B_SPLINE_CURVE ( 2, ( #3536, #13326, #15967, #17255, #6164, #726, #6250, #13232, #809 ),
 .UNSPECIFIED., .F., .T. ) 
 B_SPLINE_CURVE_WITH_KNOTS ( ( 3, 2, 2, 2, 3 ),
 ( 0.2500000000000000000, 0.2564102564102563875, 0.2692307692307692180, 0.2820512820512820484, 0.2884615384615384914 ),
 .UNSPECIFIED. ) 
 CURVE ( )  GEOMETRIC_REPRESENTATION_ITEM ( )  RATIONAL_B_SPLINE_CURVE ( ( 0.9330127018922194093, 0.9330127018922195203, 1.000000000000000000, 0.8660254037844387076, 1.000000000000000000, 0.8660254037844387076, 1.000000000000000000, 0.9330127018922190762, 0.9330127018922194093 ) ) 
 REPRESENTATION_ITEM ( '' )  );
#16508=CARTESIAN_POINT ( 'NONE',  ( 27.72904566057427189, -3.442105416578422172, -3.627061608673662896 ) ) ;
#16520=CARTESIAN_POINT ( 'NONE',  ( 28.13194630731337753, -5.901445976576172647, -3.627061608673667781 ) ) ;
#16537=CARTESIAN_POINT ( 'NONE',  ( 26.39370705969127684, -2.976016814310973313, -6.861505862736158257 ) ) ;
#16539=DIRECTION ( 'NONE',  ( 0.9928203230275512992, 0.1196152422706610041, 9.614813431917824012E-17 ) ) ;
#16542=DIRECTION ( 'NONE',  ( 0.9928203230275512992, 0.1196152422706610041, 9.614813431917824012E-17 ) ) ;
#16545=ORIENTED_EDGE ( 'NONE', *, *, #6251, .F. ) ;
#16546=CARTESIAN_POINT ( 'NONE',  ( 39.61846472826311327, -7.045996035215874365, -5.783357778048665132 ) ) ;
#16548=DIRECTION ( 'NONE',  ( 0.9928203230275512992, 0.1196152422706610180, 4.006172263299093133E-17 ) ) ;
#16557=CYLINDRICAL_SURFACE ( 'NONE', #61, 2.500000000000001776 ) ;
#16561=VERTEX_POINT ( 'NONE', #5966 ) ;
#16571=EDGE_LOOP ( 'NONE', ( #3756, #15934 ) ) ;
#16573=CARTESIAN_POINT ( 'NONE',  ( 38.97925773053390941, -7.992821573592764572, -5.783357778048662468 ) ) ;
#16575=CARTESIAN_POINT ( 'NONE',  ( 27.02867472334902033, -6.034368414549446058, -3.627061608673668225 ) ) ;
#16578=CARTESIAN_POINT ( 'NONE',  ( 29.18947247604337392, -3.066280307211263878, -8.283357778048658915 ) ) ;
#16587=CARTESIAN_POINT ( 'NONE',  ( 30.28142597461332741, -2.507623461452779701, -4.705209693361160461 ) ) ;
#16599=DIRECTION ( 'NONE',  ( 0.1196152422706608515, -0.9928203230275510771, 4.694733121053619507E-17 ) ) ;
#16601=CARTESIAN_POINT ( 'NONE',  ( 28.24571643650507369, -4.633797857156355171, -7.939653947423662039 ) ) ;
#16611=CARTESIAN_POINT ( 'NONE',  ( 26.01652455409633902, -4.902371455920926380, -5.783357778048663356 ) ) ;
#16614=CARTESIAN_POINT ( 'NONE',  ( 30.23341599105502908, -5.648260380436596506, -7.939653947423662927 ) ) ;
#16629=CARTESIAN_POINT ( 'NONE',  ( 28.41655006632555569, -6.494127376913395366, -4.705209693361169343 ) ) ;
#16642=VERTEX_POINT ( 'NONE', #11492 ) ;
#16647=CARTESIAN_POINT ( 'NONE',  ( 27.90727577511918867, -2.156494279411373061, -5.783357778048670461 ) ) ;
#16659=CARTESIAN_POINT ( 'NONE',  ( 28.84872679426759845, -7.079226011327149237, -6.453230759126474148 ) ) ;
#16663=ORIENTED_EDGE ( 'NONE', *, *, #1662, .F. ) ;
#16667=CARTESIAN_POINT ( 'NONE',  ( 33.60446413004628141, -3.988174587000466342, -3.627061608673664672 ) ) ;
#16668=PLANE ( 'NONE',  #14545 ) ;
#16669=CARTESIAN_POINT ( 'NONE',  ( 27.89118264539014547, -6.557423775948280742, -6.861505862736167138 ) ) ;
#16671=CARTESIAN_POINT ( 'NONE',  ( 28.63031693179632242, -2.406740715396564756, -4.533357778048659803 ) ) ;
#16672=CARTESIAN_POINT ( 'NONE',  ( 32.49625839967270480, -6.639770485940693412, -5.113484796970860558 ) ) ;
#16673=DIRECTION ( 'NONE',  ( -0.1196152422706599633, 0.9928203230275514102, 0.000000000000000000 ) ) ;
#16675=CARTESIAN_POINT ( 'NONE',  ( 29.36638131047866196, -1.990897739957422807, -5.783357778048658027 ) ) ;
#16678=CARTESIAN_POINT ( 'NONE',  ( 27.77288575766320378, -4.690764616287755651, -7.939653947423662039 ) ) ;
#16687=CARTESIAN_POINT ( 'NONE',  ( 29.21955148510287614, -5.970283550416647600, -3.283357778048667797 ) ) ;
#16688=CARTESIAN_POINT ( 'NONE',  ( 27.75549246765397271, -7.200742295513423485, -5.783357778048668685 ) ) ;
#16697=CARTESIAN_POINT ( 'NONE',  ( 42.32364987186199556, -2.937684895442014277, -5.783357778048662468 ) ) ;
#16698=EDGE_CURVE ( 'NONE', #6479, #7654, #6691, .T. ) ;
#16699=ORIENTED_EDGE ( 'NONE', *, *, #9447, .F. ) ;
#16701=CARTESIAN_POINT ( 'NONE',  ( 27.47505859511117521, -2.218764776483033163, -5.783357778048658915 ) ) ;
#16704=ADVANCED_FACE ( 'NONE', ( #14694 ), #5865, .T. ) ;
#16705=CARTESIAN_POINT ( 'NONE',  ( 26.01652455409633902, -4.902371455920926380, -5.783357778048663356 ) ) ;
#16709=ORIENTED_EDGE ( 'NONE', *, *, #10028, .T. ) ;
#16712=VERTEX_POINT ( 'NONE', #3325 ) ;
#16713=VECTOR ( 'NONE', #576, 1000.000000000000114 ) ;
#16718=CARTESIAN_POINT ( 'NONE',  ( 33.20111501597313719, -6.944397359513344803, -5.783357778048669573 ) ) ;
#16733=VERTEX_POINT ( 'NONE', #11553 ) ;
#16734=CARTESIAN_POINT ( 'NONE',  ( 39.16489837658902218, -5.353591089051433549, -2.283357778048670461 ) ) ;
#16743=EDGE_LOOP ( 'NONE', ( #9614, #8874, #8455, #14008 ) ) ;
#16749=ORIENTED_EDGE ( 'NONE', *, *, #1038, .T. ) ;
#16754=EDGE_CURVE ( 'NONE', #1701, #2990, #17120, .T. ) ;
#16756=CARTESIAN_POINT ( 'NONE',  ( 27.04606801335823718, -3.524390735323772006, -7.939653947423660263 ) ) ;
#16758=CARTESIAN_POINT ( 'NONE',  ( 30.69058026372202974, -5.793053633118939061, -8.283357778048662468 ) ) ;
#16762=CARTESIAN_POINT ( 'NONE',  ( 30.64918316926811315, -2.463315982128351678, -6.861505862736159145 ) ) ;
#16764=CARTESIAN_POINT ( 'NONE',  ( 26.03655646321512052, -5.068638614726478586, -8.187879365734106685 ) ) ;
#16767=ORIENTED_EDGE ( 'NONE', *, *, #13327, .T. ) ;
#16771=VERTEX_POINT ( 'NONE', #13016 ) ;
#16773=CARTESIAN_POINT ( 'NONE',  ( 28.45891156537951971, -2.090033060632186412, -5.783357778048670461 ) ) ;
#16778=CARTESIAN_POINT ( 'NONE',  ( 29.39282811755836633, -5.749534618892433002, -3.627061608673667781 ) ) ;
#16781=DIRECTION ( 'NONE',  ( 0.9928203230275510771, 0.1196152422706609902, 4.006172263299092517E-17 ) ) ;
#16790=ORIENTED_EDGE ( 'NONE', *, *, #16754, .F. ) ;
#16792=VECTOR ( 'NONE', #3108, 1000.000000000000227 ) ;
#16795=CARTESIAN_POINT ( 'NONE',  ( 29.38830135902312080, -2.615227339812091767, -6.861505862736159145 ) ) ;
#16799=FACE_OUTER_BOUND ( 'NONE', #10740, .T. ) ;
#16806=EDGE_CURVE ( 'NONE', #16322, #6149, #3555, .T. ) ;
#16815=CARTESIAN_POINT ( 'NONE',  ( 32.47301885516785092, -2.670677813450649474, -3.283357778048662023 ) ) ;
#16816=CARTESIAN_POINT ( 'NONE',  ( 31.63243098167119172, -2.771952051906466430, -8.283357778048660691 ) ) ;
#16824=ORIENTED_EDGE ( 'NONE', *, *, #15798, .F. ) ;
#16826=EDGE_CURVE ( 'NONE', #3360, #5903, #10871, .T. ) ;
#16828=CARTESIAN_POINT ( 'NONE',  ( 30.40162818048570514, -5.827866652795590241, -3.283357778048667797 ) ) ;
#16829=VECTOR ( 'NONE', #15145, 1000.000000000000227 ) ;
#16847=DIRECTION ( 'NONE',  ( 0.9928203230275512992, 0.1196152422706607682, -0.000000000000000000 ) ) ;
#16848=EDGE_LOOP ( 'NONE', ( #8597, #9525 ) ) ;
#16856=LINE ( 'NONE', #8404, #7630 ) ;
#16858=CARTESIAN_POINT ( 'NONE',  ( 29.35841309260160159, -6.680460261459264970, -4.533357778048668685 ) ) ;
#16859=CARTESIAN_POINT ( 'NONE',  ( 33.18226487515251932, -2.585227674546096477, -3.283357778048662023 ) ) ;
#16862=CARTESIAN_POINT ( 'NONE',  ( 32.77709966008947617, -5.968767264923789284, -6.861505862736166250 ) ) ;
#16865=CARTESIAN_POINT ( 'NONE',  ( 25.76466184735054910, -2.811881907026620553, -6.248149982130924762 ) ) ;
#16866=CARTESIAN_POINT ( 'NONE',  ( 27.45273115869273539, -7.247415916675651992, -5.113484796970856117 ) ) ;
#16867=AXIS2_PLACEMENT_3D ( 'NONE', #15056, #10948, #5607 ) ;
#16874=AXIS2_PLACEMENT_3D ( 'NONE', #3967, #13668, #8306 ) ;
#16875=CARTESIAN_POINT ( 'NONE',  ( 25.29083129957448151, -4.989803161779970964, -5.783357778048664244 ) ) ;
#16879=CARTESIAN_POINT ( 'NONE',  ( 31.41531425212677675, -1.744041783721344219, -5.783357778048658027 ) ) ;
#16882=CONICAL_SURFACE ( 'NONE', #2117, 3.500000000000004885, 0.1745329251994333364 ) ;
#16896=CARTESIAN_POINT ( 'NONE',  ( 26.47269060886452507, -6.728324053342490174, -6.861505862736166250 ) ) ;
#16897=VERTEX_POINT ( 'NONE', #5532 ) ;
#16900=CARTESIAN_POINT ( 'NONE',  ( 26.92924972366625980, -7.310485091653801781, -5.783357778048657138 ) ) ;
#16913=CARTESIAN_POINT ( 'NONE',  ( 31.70371634254663817, -2.036456781249897485, -4.533357778048659803 ) ) ;
#16925=CARTESIAN_POINT ( 'NONE',  ( 26.01652455409633902, -4.902371455920926380, -5.783357778048663356 ) ) ;
#16927=FACE_OUTER_BOUND ( 'NONE', #17032, .T. ) ;
#16932=CARTESIAN_POINT ( 'NONE',  ( 32.18597209352066812, -4.159074864394664672, -7.939653947423662039 ) ) ;
#16934=CYLINDRICAL_SURFACE ( 'NONE', #6319, 2.500000000000001776 ) ;
#16940=CARTESIAN_POINT ( 'NONE',  ( 31.94462260941237020, -6.706231704719880504, -5.113484796970860558 ) ) ;
#16942=EDGE_CURVE ( 'NONE', #8853, #15406, #9122, .T. ) ;
#16949=DIRECTION ( 'NONE',  ( 0.9928203230275510771, 0.1196152422706609902, 4.006172263299092517E-17 ) ) ;
#16950=CARTESIAN_POINT ( 'NONE',  ( 26.34507017448785504, -7.770415366711231009, -5.783357778048669573 ) ) ;
#16952=CARTESIAN_POINT ( 'NONE',  ( 32.95080301609915097, -1.548848848676412260, -5.783357778048662468 ) ) ;
#16955=CARTESIAN_POINT ( 'NONE',  ( 32.12473870642251939, -5.420393343910986594, -7.939653947423664704 ) ) ;
#16956=CARTESIAN_POINT ( 'NONE',  ( 26.51200394741821498, -4.842675973971495296, -7.939653947423662039 ) ) ;
#16957=CARTESIAN_POINT ( 'NONE',  ( 26.59574320524588842, -2.314508053356755024, -5.113484796970857893 ) ) ;
#16967=CARTESIAN_POINT ( 'NONE',  ( 31.56875459193803124, -6.114348982704044921, -4.705209693361169343 ) ) ;
#16981=CYLINDRICAL_SURFACE ( 'NONE', #4260, 2.500000000000001776 ) ;
#16989=( BOUNDED_CURVE ( )  B_SPLINE_CURVE ( 2, ( #887, #8955, #2436, #11937, #711, #11671, #14499, #10650, #12024 ),
 .UNSPECIFIED., .F., .T. ) 
 B_SPLINE_CURVE_WITH_KNOTS ( ( 3, 2, 2, 2, 3 ),
 ( 0.1346153846153846367, 0.1410256410256410242, 0.1538461538461538547, 0.1666666666666666574, 0.1730769230769231004 ),
 .UNSPECIFIED. ) 
 CURVE ( )  GEOMETRIC_REPRESENTATION_ITEM ( )  RATIONAL_B_SPLINE_CURVE ( ( 0.9330127018922194093, 0.9330127018922196314, 1.000000000000000000, 0.8660254037844387076, 1.000000000000000000, 0.8660254037844387076, 1.000000000000000000, 0.9330127018922190762, 0.9330127018922194093 ) ) 
 REPRESENTATION_ITEM ( '' )  );
#16991=ADVANCED_FACE ( 'NONE', ( #1567 ), #15705, .T. ) ;
#16996=CARTESIAN_POINT ( 'NONE',  ( 33.95908713831674675, -3.945449517755637903, -5.783357778048663356 ) ) ;
#16997=VERTEX_POINT ( 'NONE', #14349 ) ;
#16998=CARTESIAN_POINT ( 'NONE',  ( 33.01342578063301403, -4.059383036018435753, -8.283357778048662468 ) ) ;
#17006=ORIENTED_EDGE ( 'NONE', *, *, #12395, .T. ) ;
#17012=ORIENTED_EDGE ( 'NONE', *, *, #10188, .T. ) ;
#17021=CARTESIAN_POINT ( 'NONE',  ( 33.43363050022580296, -2.127845067243429256, -4.705209693361160461 ) ) ;
#17022=CARTESIAN_POINT ( 'NONE',  ( 41.90164972253718645, -2.988527579590353422, -5.783357778048662468 ) ) ;
#17027=CARTESIAN_POINT ( 'NONE',  ( 26.35439372113758694, -4.861664893681965083, -7.939653947423662039 ) ) ;
#17032=EDGE_LOOP ( 'NONE', ( #2679, #9852, #14338, #2241 ) ) ;
#17036=CARTESIAN_POINT ( 'NONE',  ( 27.73348320195396965, -4.695511846111656062, -3.283357778048664688 ) ) ;
#17042=CARTESIAN_POINT ( 'NONE',  ( 31.91459173804834748, -5.445711903524953712, -3.627061608673667781 ) ) ;
#17044=ADVANCED_FACE ( 'NONE', ( #11223 ), #1934, .T. ) ;
#17058=CARTESIAN_POINT ( 'NONE',  ( 31.03886041246737548, -3.043338102658604161, -3.627061608673662008 ) ) ;
#17059=CARTESIAN_POINT ( 'NONE',  ( 29.98885399772409954, -6.604504582617394703, -4.533357778048668685 ) ) ;
#17060=CARTESIAN_POINT ( 'NONE',  ( 27.57216386142120257, -6.895668018177890879, -7.033357778048666908 ) ) ;
#17062=ADVANCED_FACE ( 'NONE', ( #16799 ), #111, .F. ) ;
#17070=CARTESIAN_POINT ( 'NONE',  ( 33.40660799972355477, 0.6401911282994665608, -5.783357778048661579 ) ) ;
#17072=LINE ( 'NONE', #13877, #10073 ) ;
#17074=CARTESIAN_POINT ( 'NONE',  ( 26.23609683341064525, -2.995005734021441768, -6.861505862736159145 ) ) ;
#17083=CARTESIAN_POINT ( 'NONE',  ( 26.53943449477818106, -2.321292140958837624, -6.453230759126469707 ) ) ;
#17088=CARTESIAN_POINT ( 'NONE',  ( 28.55151181693415907, -2.416235175459247486, -4.533357778048659803 ) ) ;
#17091=CARTESIAN_POINT ( 'NONE',  ( 30.54048978798443059, -6.538043363838207611, -4.533357778048668685 ) ) ;
#17097=( BOUNDED_CURVE ( )  B_SPLINE_CURVE ( 2, ( #2023, #10520, #13437, #2120, #9252, #11788, #14712, #17461, #2294 ),
 .UNSPECIFIED., .F., .T. ) 
 B_SPLINE_CURVE_WITH_KNOTS ( ( 3, 2, 2, 2, 3 ),
 ( 0.6730769230769231282, 0.6794871794871795156, 0.6923076923076922906, 0.7051282051282051766, 0.7115384615384615641 ),
 .UNSPECIFIED. ) 
 CURVE ( )  GEOMETRIC_REPRESENTATION_ITEM ( )  RATIONAL_B_SPLINE_CURVE ( ( 0.9330127018922192983, 0.9330127018922198534, 1.000000000000000000, 0.8660254037844387076, 1.000000000000000000, 0.8660254037844387076, 1.000000000000000000, 0.9330127018922194093, 0.9330127018922194093 ) ) 
 REPRESENTATION_ITEM ( '' )  );
#17108=DIRECTION ( 'NONE',  ( -0.1196152422706610735, 0.9928203230275511881, 0.000000000000000000 ) ) ;
#17109=CARTESIAN_POINT ( 'NONE',  ( 26.01652455409633902, -4.902371455920926380, -5.783357778048663356 ) ) ;
#17113=CARTESIAN_POINT ( 'NONE',  ( 32.30426898124760982, -6.025734024055190652, -6.861505862736167138 ) ) ;
#17120=LINE ( 'NONE', #15749, #988 ) ;
#17132=CARTESIAN_POINT ( 'NONE',  ( 29.16815758536418102, -2.004582921727632971, -5.783357778048664244 ) ) ;
#17135=CARTESIAN_POINT ( 'NONE',  ( 27.26436163736424945, -2.571311352887278190, -7.033357778048658027 ) ) ;
#17139=CARTESIAN_POINT ( 'NONE',  ( 26.87106449706838873, -6.053357334259913181, -3.627061608673667781 ) ) ;
#17153=CARTESIAN_POINT ( 'NONE',  ( 30.78487334700428590, -1.819997462563214263, -5.783357778048658027 ) ) ;
#17156=ADVANCED_FACE ( 'NONE', ( #8601 ), #2892, .F. ) ;
#17157=CARTESIAN_POINT ( 'NONE',  ( 41.90164972253716513, -2.988527579590351646, -5.783357778048662468 ) ) ;
#17162=EDGE_LOOP ( 'NONE', ( #15578, #9166, #1524, #1832 ) ) ;
#17166=CARTESIAN_POINT ( 'NONE',  ( 26.01652455409633902, -4.902371455920926380, -5.783357778048663356 ) ) ;
#17168=ADVANCED_FACE ( 'NONE', ( #15584, #13957 ), #12771, .T. ) ;
#17174=CIRCLE ( 'NONE', #2118, 0.9999999999999995559 ) ;
#17187=CARTESIAN_POINT ( 'NONE',  ( 29.07687923786957285, -2.352938776424351008, -7.033357778048658027 ) ) ;
#17188=B_SPLINE_CURVE_WITH_KNOTS ( 'NONE', 1,
 ( #1911, #1637 ),
 .UNSPECIFIED., .F., .F.,
 ( 2, 2 ),
 ( 0.000000000000000000, 1.000000000000000000 ),
 .UNSPECIFIED. ) ;
#17192=VERTEX_POINT ( 'NONE', #16773 ) ;
#17200=CARTESIAN_POINT ( 'NONE',  ( 33.86058074732183343, -3.957317592522819005, -3.455209693361164902 ) ) ;
#17201=VERTEX_POINT ( 'NONE', #11399 ) ;
#17202=CARTESIAN_POINT ( 'NONE',  ( 25.76466184735054910, -2.811881907026620553, -6.248149982130924762 ) ) ;
#17203=CARTESIAN_POINT ( 'NONE',  ( 26.25597102934084859, -6.889804849753313754, -7.289619350601861392 ) ) ;
#17204=CARTESIAN_POINT ( 'NONE',  ( 33.95908713831674675, -3.945449517755637903, -5.783357778048663356 ) ) ;
#17210=DIRECTION ( 'NONE',  ( -0.1196152422706610041, 0.9928203230275510771, 0.000000000000000000 ) ) ;
#17212=CARTESIAN_POINT ( 'NONE',  ( 33.54323074294813267, -5.249493066516778050, -7.939653947423664704 ) ) ;
#17218=ORIENTED_EDGE ( 'NONE', *, *, #829, .F. ) ;
#17219=CARTESIAN_POINT ( 'NONE',  ( 26.86653773853314320, -2.919050055179571945, -6.861505862736159145 ) ) ;
#17226=DIRECTION ( 'NONE',  ( -0.1035898384862230653, 0.8598076211353318232, -0.4999999999999999445 ) ) ;
#17231=CARTESIAN_POINT ( 'NONE',  ( 26.60013260893011378, -1.924431040879551746, -5.783357778048658027 ) ) ;
#17236=CARTESIAN_POINT ( 'NONE',  ( 28.99445422935450267, -6.424501337975009996, -6.861505862736166250 ) ) ;
#17251=CARTESIAN_POINT ( 'NONE',  ( 32.28234893270314387, -5.401404424200516807, -7.939653947423664704 ) ) ;
#17252=LINE ( 'NONE', #3532, #12483 ) ;
#17255=CARTESIAN_POINT ( 'NONE',  ( 31.08079519141086067, -2.838413270685653078, -8.283357778048660691 ) ) ;
#17258=VERTEX_POINT ( 'NONE', #17535 ) ;
#17280=CARTESIAN_POINT ( 'NONE',  ( 29.77118727536320719, -5.903822331637461396, -3.283357778048667797 ) ) ;
#17291=CARTESIAN_POINT ( 'NONE',  ( 25.94006848055682113, -4.267777217026356595, -3.719179227265282162 ) ) ;
#17300=CARTESIAN_POINT ( 'NONE',  ( 29.97942892559193950, -4.424919740341219487, -3.627061608673664672 ) ) ;
#17308=CARTESIAN_POINT ( 'NONE',  ( 25.81099976294218479, -6.186279776075334524, -7.540300355390971987 ) ) ;
#17317=CARTESIAN_POINT ( 'NONE',  ( 30.64918316926811315, -2.463315982128351678, -6.861505862736159145 ) ) ;
#17319=FACE_OUTER_BOUND ( 'NONE', #9258, .T. ) ;
#17321=CARTESIAN_POINT ( 'NONE',  ( 27.47505859511117521, -2.218764776483033163, -5.783357778048658027 ) ) ;
#17322=( BOUNDED_CURVE ( )  B_SPLINE_CURVE ( 2, ( #11586, #902, #10500, #2001, #17539, #3352, #7620, #16061, #9153 ),
 .UNSPECIFIED., .F., .T. ) 
 B_SPLINE_CURVE_WITH_KNOTS ( ( 3, 2, 2, 2, 3 ),
 ( 0.4038461538461538547, 0.4102564102564102422, 0.4230769230769230727, 0.4358974358974359031, 0.4423076923076923461 ),
 .UNSPECIFIED. ) 
 CURVE ( )  GEOMETRIC_REPRESENTATION_ITEM ( )  RATIONAL_B_SPLINE_CURVE ( ( 0.9330127018922194093, 0.9330127018922196314, 1.000000000000000000, 0.8660254037844387076, 1.000000000000000000, 0.8660254037844387076, 1.000000000000000000, 0.9330127018922190762, 0.9330127018922194093 ) ) 
 REPRESENTATION_ITEM ( '' )  );
#17328=ORIENTED_EDGE ( 'NONE', *, *, #8089, .F. ) ;
#17340=CARTESIAN_POINT ( 'NONE',  ( 27.67650891848073158, -3.448435056481901295, -7.939653947423660263 ) ) ;
#17342=FACE_OUTER_BOUND ( 'NONE', #10630, .T. ) ;
#17344=CARTESIAN_POINT ( 'NONE',  ( 38.15053902264412500, -1.114360604510108876, -1.783357778048662912 ) ) ;
#17350=CARTESIAN_POINT ( 'NONE',  ( 32.07220196432898263, -5.426722983814484813, -3.627061608673668225 ) ) ;
#17368=VECTOR ( 'NONE', #14761, 1000.000000000000114 ) ;
#17377=CARTESIAN_POINT ( 'NONE',  ( 30.01512236704901682, -6.601339762873093875, -7.033357778048666908 ) ) ;
#17378=CARTESIAN_POINT ( 'NONE',  ( 31.53813789838894621, -6.745008222462202774, -5.783357778048668685 ) ) ;
#17382=CARTESIAN_POINT ( 'NONE',  ( 26.94172295629870462, -6.971623697019761146, -7.033357778048666908 ) ) ;
#17389=CARTESIAN_POINT ( 'NONE',  ( 25.75668387115780078, -2.745663783273349257, -5.690028976746116740 ) ) ;
#17399=CARTESIAN_POINT ( 'NONE',  ( 31.54230778485832332, -2.355712103769039611, -4.705209693361160461 ) ) ;
#17414=CARTESIAN_POINT ( 'NONE',  ( 26.31137250323187260, -7.349643480353759806, -6.203850694058635540 ) ) ;
#17417=CARTESIAN_POINT ( 'NONE',  ( 32.02836186724004364, -4.178063784105134459, -7.939653947423662039 ) ) ;
#17419=CARTESIAN_POINT ( 'NONE',  ( 31.68992120585416217, -1.700760206360153015, -5.783357778048664244 ) ) ;
#17420=CARTESIAN_POINT ( 'NONE',  ( 28.14933959732260149, -3.391468297350501260, -7.939653947423660263 ) ) ;
#17439=CARTESIAN_POINT ( 'NONE',  ( 29.54591158530375239, -2.596238420101622868, -6.861505862736158257 ) ) ;
#17442=CARTESIAN_POINT ( 'NONE',  ( 31.64365984991007252, -1.316785610144591390, -5.783357778048658027 ) ) ;
#17448=CARTESIAN_POINT ( 'NONE',  ( 31.56875459193803124, -6.114348982704044921, -4.705209693361169343 ) ) ;
#17461=CARTESIAN_POINT ( 'NONE',  ( 27.85662501549087366, -2.162596695673018043, -5.113484796970851676 ) ) ;
#17462=EDGE_LOOP ( 'NONE', ( #6285, #16663, #13017, #15973 ) ) ;
#17469=CARTESIAN_POINT ( 'NONE',  ( 26.06962060539356330, -5.343074812781621219, -3.590724507760069795 ) ) ;
#17473=CARTESIAN_POINT ( 'NONE',  ( 28.09001152836989235, -6.106370808549102414, -8.283357778048662468 ) ) ;
#17474=CARTESIAN_POINT ( 'NONE',  ( 30.62726312072365431, -1.838986382273682718, -5.783357778048658915 ) ) ;
#17482=CARTESIAN_POINT ( 'NONE',  ( 30.48043329534786849, -5.818372192732907067, -3.283357778048667797 ) ) ;
#17484=VERTEX_POINT ( 'NONE', #17681 ) ;
#17488=DIRECTION ( 'NONE',  ( 0.000000000000000000, 1.000000000000000000, -4.661026453772598353E-17 ) ) ;
#17495=EDGE_CURVE ( 'NONE', #2702, #8269, #12286, .T. ) ;
#17499=CARTESIAN_POINT ( 'NONE',  ( 31.43723430067123914, -2.368371383576012956, -6.861505862736158257 ) ) ;
#17506=STYLED_ITEM ( 'NONE', ( #8559 ), #17610 ) ;
#17507=ORIENTED_EDGE ( 'NONE', *, *, #11187, .F. ) ;
#17514=PLANE ( 'NONE',  #9264 ) ;
#17515=CARTESIAN_POINT ( 'NONE',  ( 41.60261161686052134, -0.5064767720214741198, -5.783357778048662468 ) ) ;
#17518=CARTESIAN_POINT ( 'NONE',  ( 30.88125018618674744, -3.062327022369072171, -3.627061608673662896 ) ) ;
#17523=CARTESIAN_POINT ( 'NONE',  ( 26.86653773853314320, -2.919050055179571945, -6.861505862736159145 ) ) ;
#17531=EDGE_CURVE ( 'NONE', #6798, #14747, #9462, .T. ) ;
#17535=CARTESIAN_POINT ( 'NONE',  ( 31.97277696464621854, -6.702839660918840536, -5.783357778048663356 ) ) ;
#17538=CARTESIAN_POINT ( 'NONE',  ( 29.78250536075762867, -6.329556739422670830, -6.861505862736167138 ) ) ;
#17539=CARTESIAN_POINT ( 'NONE',  ( 30.49166216014303643, -4.363205751385915931, -8.283357778048662468 ) ) ;
#17542=CARTESIAN_POINT ( 'NONE',  ( 26.56758885001203652, -2.317900097157796324, -5.783357778048670461 ) ) ;
#17545=VECTOR ( 'NONE', #17746, 1000.000000000000114 ) ;
#17547=CARTESIAN_POINT ( 'NONE',  ( 33.30663696749426350, -1.516174747195734085, -5.783357778048658915 ) ) ;
#17548=VERTEX_POINT ( 'NONE', #1234 ) ;
#17549=FACE_OUTER_BOUND ( 'NONE', #11221, .T. ) ;
#17552=PRODUCT_DEFINITION_SHAPE ( 'NONE', 'NONE',  #14992 ) ;
#17556=ORIENTED_EDGE ( 'NONE', *, *, #12700, .F. ) ;
#17557=EDGE_CURVE ( 'NONE', #2500, #12046, #17627, .T. ) ;
#17561=CARTESIAN_POINT ( 'NONE',  ( 29.74110826630371207, -2.999819088432076786, -8.283357778048660691 ) ) ;
#17565=CARTESIAN_POINT ( 'NONE',  ( 26.31176419598820360, -7.352894575460818594, -6.182016197336221985 ) ) ;
#17568=CARTESIAN_POINT ( 'NONE',  ( 29.86122125502053848, -4.439161430227785310, -8.283357778048662468 ) ) ;
#17569=CARTESIAN_POINT ( 'NONE',  ( 32.54050588463559990, -2.235448945602741766, -6.861505862736159145 ) ) ;
#17573=CARTESIAN_POINT ( 'NONE',  ( 26.61823960964035507, -2.311797680896151341, -6.453230759126464378 ) ) ;
#17575=DIRECTION ( 'NONE',  ( 0.000000000000000000, 0.000000000000000000, 1.000000000000000000 ) ) ;
#17584=VERTEX_POINT ( 'NONE', #5555 ) ;
#17585=CARTESIAN_POINT ( 'NONE',  ( 28.28502977505876359, -2.748149777785362957, -6.861505862736158257 ) ) ;
#17586=CARTESIAN_POINT ( 'NONE',  ( 33.14902674121363901, -1.535163666906202318, -5.783357778048658027 ) ) ;
#17596=CARTESIAN_POINT ( 'NONE',  ( 33.13353876934985465, -5.498725377814142057, -8.283357778048664244 ) ) ;
#17601=( BOUNDED_CURVE ( )  B_SPLINE_CURVE ( 2, ( #379, #1734, #12878, #10316, #8889, #14423, #14058, #7532, #7264 ),
 .UNSPECIFIED., .F., .T. ) 
 B_SPLINE_CURVE_WITH_KNOTS ( ( 3, 2, 2, 2, 3 ),
 ( 0.7115384615384615641, 0.7179487179487179516, 0.7307692307692307265, 0.7435897435897436125, 0.7500000000000000000 ),
 .UNSPECIFIED. ) 
 CURVE ( )  GEOMETRIC_REPRESENTATION_ITEM ( )  RATIONAL_B_SPLINE_CURVE ( ( 0.9330127018922194093, 0.9330127018922194093, 1.000000000000000000, 0.8660254037844387076, 1.000000000000000000, 0.8660254037844387076, 1.000000000000000000, 0.9330127018922194093, 0.9330127018922194093 ) ) 
 REPRESENTATION_ITEM ( '' )  );
#17602=CARTESIAN_POINT ( 'NONE',  ( 31.39792096211754924, -4.254019462947003838, -7.939653947423662039 ) ) ;
#17606=( BOUNDED_CURVE ( )  B_SPLINE_CURVE ( 2, ( #16900, #17642, #5250, #12416, #17818, #4181, #1363, #5161, #2467 ),
 .UNSPECIFIED., .F., .T. ) 
 B_SPLINE_CURVE_WITH_KNOTS ( ( 3, 2, 2, 2, 3 ),
 ( 0.8269230769230769829, 0.8333333333333333703, 0.8461538461538461453, 0.8589743589743589203, 0.8653846153846154188 ),
 .UNSPECIFIED. ) 
 CURVE ( )  GEOMETRIC_REPRESENTATION_ITEM ( )  RATIONAL_B_SPLINE_CURVE ( ( 0.9330127018922192983, 0.9330127018922198534, 1.000000000000000000, 0.8660254037844387076, 1.000000000000000000, 0.8660254037844387076, 1.000000000000000000, 0.9330127018922187432, 0.9330127018922192983 ) ) 
 REPRESENTATION_ITEM ( '' )  );
#17610=MANIFOLD_SOLID_BREP ( 'Cavity1', #12740 ) ;
#17619=CARTESIAN_POINT ( 'NONE',  ( 31.12210306526553083, -4.287250072544045665, -8.283357778048662468 ) ) ;
#17621=CARTESIAN_POINT ( 'NONE',  ( 29.94002636988270538, -4.429666970165102136, -8.283357778048662468 ) ) ;
#17623=CARTESIAN_POINT ( 'NONE',  ( 30.80679339554874119, -2.444327062417882779, -6.861505862736158257 ) ) ;
#17627=( BOUNDED_CURVE ( )  B_SPLINE_CURVE ( 2, ( #14752, #12013, #13293, #873, #11924, #17596, #10635, #3774, #2422 ),
 .UNSPECIFIED., .F., .T. ) 
 B_SPLINE_CURVE_WITH_KNOTS ( ( 3, 2, 2, 2, 3 ),
 ( 0.09615384615384617306, 0.1025641025641025605, 0.1153846153846153910, 0.1282051282051281937, 0.1346153846153846367 ),
 .UNSPECIFIED. ) 
 CURVE ( )  GEOMETRIC_REPRESENTATION_ITEM ( )  RATIONAL_B_SPLINE_CURVE ( ( 0.9330127018922194093, 0.9330127018922196314, 1.000000000000000000, 0.8660254037844387076, 1.000000000000000000, 0.8660254037844387076, 1.000000000000000000, 0.9330127018922190762, 0.9330127018922194093 ) ) 
 REPRESENTATION_ITEM ( '' )  );
#17632=CARTESIAN_POINT ( 'NONE',  ( 30.93831368681553684, -6.190304661545915188, -4.705209693361169343 ) ) ;
#17642=CARTESIAN_POINT ( 'NONE',  ( 26.90109536843240789, -7.313877135454839973, -5.113484796970856117 ) ) ;
#17649=CARTESIAN_POINT ( 'NONE',  ( 26.23123039439649062, -6.684454722870800225, -4.255767710538254534 ) ) ;
#17651=CARTESIAN_POINT ( 'NONE',  ( 26.75784435724945709, -6.993777436889428323, -4.533357778048668685 ) ) ;
#17652=CARTESIAN_POINT ( 'NONE',  ( 30.45225960443380231, -4.367952981209816343, -3.627061608673664672 ) ) ;
#17653=VECTOR ( 'NONE', #4006, 1000.000000000000114 ) ;
#17666=CARTESIAN_POINT ( 'NONE',  ( 25.71748644841968456, -2.420320648352046078, -5.783357778048663356 ) ) ;
#17669=CARTESIAN_POINT ( 'NONE',  ( 26.01127209431523113, -6.877383572197488526, -7.035051132944705188 ) ) ;
#17671=EDGE_CURVE ( 'NONE', #13726, #757, #6004, .T. ) ;
#17681=CARTESIAN_POINT ( 'NONE',  ( 38.68147913031998542, -1.341155523753224887, -9.283357778048653586 ) ) ;
#17683=CARTESIAN_POINT ( 'NONE',  ( 26.01652455409633902, -4.902371455920926380, -5.783357778048663356 ) ) ;
#17685=CARTESIAN_POINT ( 'NONE',  ( 26.31176419598820360, -7.352894575460818594, -6.182016197336221985 ) ) ;
#17705=( BOUNDED_CURVE ( )  B_SPLINE_CURVE ( 2, ( #4584, #1889, #6027, #12845, #435, #150, #12928, #5939, #12654 ),
 .UNSPECIFIED., .F., .T. ) 
 B_SPLINE_CURVE_WITH_KNOTS ( ( 3, 2, 2, 2, 3 ),
 ( 0.1346153846153846367, 0.1410256410256410242, 0.1538461538461538547, 0.1666666666666666574, 0.1730769230769231004 ),
 .UNSPECIFIED. ) 
 CURVE ( )  GEOMETRIC_REPRESENTATION_ITEM ( )  RATIONAL_B_SPLINE_CURVE ( ( 0.9330127018922194093, 0.9330127018922196314, 1.000000000000000000, 0.8660254037844387076, 1.000000000000000000, 0.8660254037844387076, 1.000000000000000000, 0.9330127018922190762, 0.9330127018922194093 ) ) 
 REPRESENTATION_ITEM ( '' )  );
#17709=CARTESIAN_POINT ( 'NONE',  ( 29.67743187657054449, -6.342216019229654833, -4.705209693361169343 ) ) ;
#17719=CARTESIAN_POINT ( 'NONE',  ( 33.13163345120441505, -4.045141346131868154, -3.627061608673664672 ) ) ;
#17723=VERTEX_POINT ( 'NONE', #7475 ) ;
#17728=( BOUNDED_CURVE ( )  B_SPLINE_CURVE ( 2, ( #11130, #14149, #2818, #1561, #8346, #8439, #14067, #13974, #9776 ),
 .UNSPECIFIED., .F., .T. ) 
 B_SPLINE_CURVE_WITH_KNOTS ( ( 3, 2, 2, 2, 3 ),
 ( 0.3653846153846154188, 0.3717948717948718063, 0.3846153846153846367, 0.3974358974358974117, 0.4038461538461538547 ),
 .UNSPECIFIED. ) 
 CURVE ( )  GEOMETRIC_REPRESENTATION_ITEM ( )  RATIONAL_B_SPLINE_CURVE ( ( 0.9330127018922194093, 0.9330127018922196314, 1.000000000000000000, 0.8660254037844387076, 1.000000000000000000, 0.8660254037844387076, 1.000000000000000000, 0.9330127018922190762, 0.9330127018922194093 ) ) 
 REPRESENTATION_ITEM ( '' )  );
#17729=DIRECTION ( 'NONE',  ( 0.9928203230275512992, 0.1196152422706610041, 9.614813431917824012E-17 ) ) ;
#17730=CARTESIAN_POINT ( 'NONE',  ( 28.45891156537951971, -2.090033060632186412, -5.783357778048670461 ) ) ;
#17740=CARTESIAN_POINT ( 'NONE',  ( 33.78529456515154550, -6.484467084455914687, -5.783357778048663356 ) ) ;
#17743=EDGE_CURVE ( 'NONE', #17723, #627, #3481, .T. ) ;
#17744=CARTESIAN_POINT ( 'NONE',  ( 33.17094678975809074, -2.159493266760871499, -6.861505862736159145 ) ) ;
#17746=DIRECTION ( 'NONE',  ( 0.1196152422706609625, -0.9928203230275510771, 4.694733121053620740E-17 ) ) ;
#17755=VECTOR ( 'NONE', #3777, 999.9999999999998863 ) ;
#17757=CARTESIAN_POINT ( 'NONE',  ( 28.49970350196817392, -5.857138497251738407, -7.939653947423664704 ) ) ;
#17767=ORIENTED_EDGE ( 'NONE', *, *, #15431, .F. ) ;
#17771=AXIS2_PLACEMENT_3D ( 'NONE', #2526, #8054, #6786 ) ;
#17783=DIRECTION ( 'NONE',  ( 0.9928203230275512992, 0.1196152422706610180, 4.006172263299093133E-17 ) ) ;
#17788=ORIENTED_EDGE ( 'NONE', *, *, #14348, .T. ) ;
#17794=DIRECTION ( 'NONE',  ( -0.9928203230275512992, -0.1196152422706610180, -9.614813431917824012E-17 ) ) ;
#17795=CARTESIAN_POINT ( 'NONE',  ( 33.76207435632690590, -3.969185667289998332, -3.627061608673664672 ) ) ;
#17796=ADVANCED_FACE ( 'NONE', ( #1868 ), #7659, .F. ) ;
#17798=CARTESIAN_POINT ( 'NONE',  ( 26.39370705969127684, -2.976016814310973313, -6.861505862736158257 ) ) ;
#17807=CARTESIAN_POINT ( 'NONE',  ( 29.97942892559193950, -4.424919740341219487, -3.627061608673664672 ) ) ;
#17818=CARTESIAN_POINT ( 'NONE',  ( 26.47260139170898441, -4.847423203795396596, -3.283357778048664688 ) ) ;
#17828=CARTESIAN_POINT ( 'NONE',  ( 26.02974819644417792, -2.720057890826728109, -4.533357778048659803 ) ) ;
#17829=CARTESIAN_POINT ( 'NONE',  ( 28.12741954877813555, -2.767138697495831856, -6.861505862736159145 ) ) ;
#17831=( BOUNDED_CURVE ( )  B_SPLINE_CURVE ( 2, ( #7479, #9996, #3125, #16828, #323, #3216, #588, #3041, #8658 ),
 .UNSPECIFIED., .F., .T. ) 
 B_SPLINE_CURVE_WITH_KNOTS ( ( 3, 2, 2, 2, 3 ),
 ( 0.4423076923076923461, 0.4487179487179487336, 0.4615384615384615641, 0.4743589743589743390, 0.4807692307692307820 ),
 .UNSPECIFIED. ) 
 CURVE ( )  GEOMETRIC_REPRESENTATION_ITEM ( )  RATIONAL_B_SPLINE_CURVE ( ( 0.9330127018922194093, 0.9330127018922196314, 1.000000000000000000, 0.8660254037844387076, 1.000000000000000000, 0.8660254037844387076, 1.000000000000000000, 0.9330127018922190762, 0.9330127018922194093 ) ) 
 REPRESENTATION_ITEM ( '' )  );
#17833=CARTESIAN_POINT ( 'NONE',  ( 42.32030307048450624, -6.463398710186787355, -5.783357778048662468 ) ) ;
#17846=CARTESIAN_POINT ( 'NONE',  ( 33.95908713831676096, -3.945449517755638791, -3.283357778048664688 ) ) ;
#17868=CARTESIAN_POINT ( 'NONE',  ( 42.20068782821381603, -5.470578387159230616, -5.783357778048662468 ) ) ;
#17875=CARTESIAN_POINT ( 'NONE',  ( 30.96820195323705605, -2.125071739898741097, -7.033357778048658027 ) ) ;
#17879=CARTESIAN_POINT ( 'NONE',  ( 26.82722439997946395, -4.804698134550569044, -3.627061608673664672 ) ) ;
#17881=CARTESIAN_POINT ( 'NONE',  ( 31.04700706809921940, -2.115577279836057922, -7.033357778048658027 ) ) ;
#17882=FACE_OUTER_BOUND ( 'NONE', #15220, .T. ) ;
#17887=CARTESIAN_POINT ( 'NONE',  ( 30.41294626588012306, -6.253601060580800564, -6.861505862736167138 ) ) ;
#17889=EDGE_CURVE ( 'NONE', #7654, #15926, #5548, .T. ) ;
#17896=CARTESIAN_POINT ( 'NONE',  ( 29.64681518302145591, -6.972875258987813574, -5.783357778048668685 ) ) ;
#17907=VERTEX_POINT ( 'NONE', #5013 ) ;
#17908=CARTESIAN_POINT ( 'NONE',  ( 26.82912971812490355, -6.258282166232842947, -8.283357778048662468 ) ) ;
#17910=CARTESIAN_POINT ( 'NONE',  ( 28.23249303296521617, -2.754479417688857179, -4.705209693361161349 ) ) ;
#17915=ORIENTED_EDGE ( 'NONE', *, *, #11504, .F. ) ;
#17924=CARTESIAN_POINT ( 'NONE',  ( 27.65458886993626564, -2.824105456627233224, -6.861505862736158257 ) ) ;
#17925=ORIENTED_EDGE ( 'NONE', *, *, #5679, .F. ) ;
#17935=CARTESIAN_POINT ( 'NONE',  ( 28.08317206381523334, -7.171460237833785278, -5.113484796970862334 ) ) ;
#17940=CARTESIAN_POINT ( 'NONE',  ( 28.72797218747911074, -6.756415940301135237, -4.533357778048668685 ) ) ;
#17960=CARTESIAN_POINT ( 'NONE',  ( 27.26074174026764751, -6.633379454790151009, -6.861505862736167138 ) ) ;
#17963=CARTESIAN_POINT ( 'NONE',  ( 30.09392748191118017, -6.591845302810410701, -7.033357778048666908 ) ) ;
ENDSEC;
END-ISO-10303-21;
